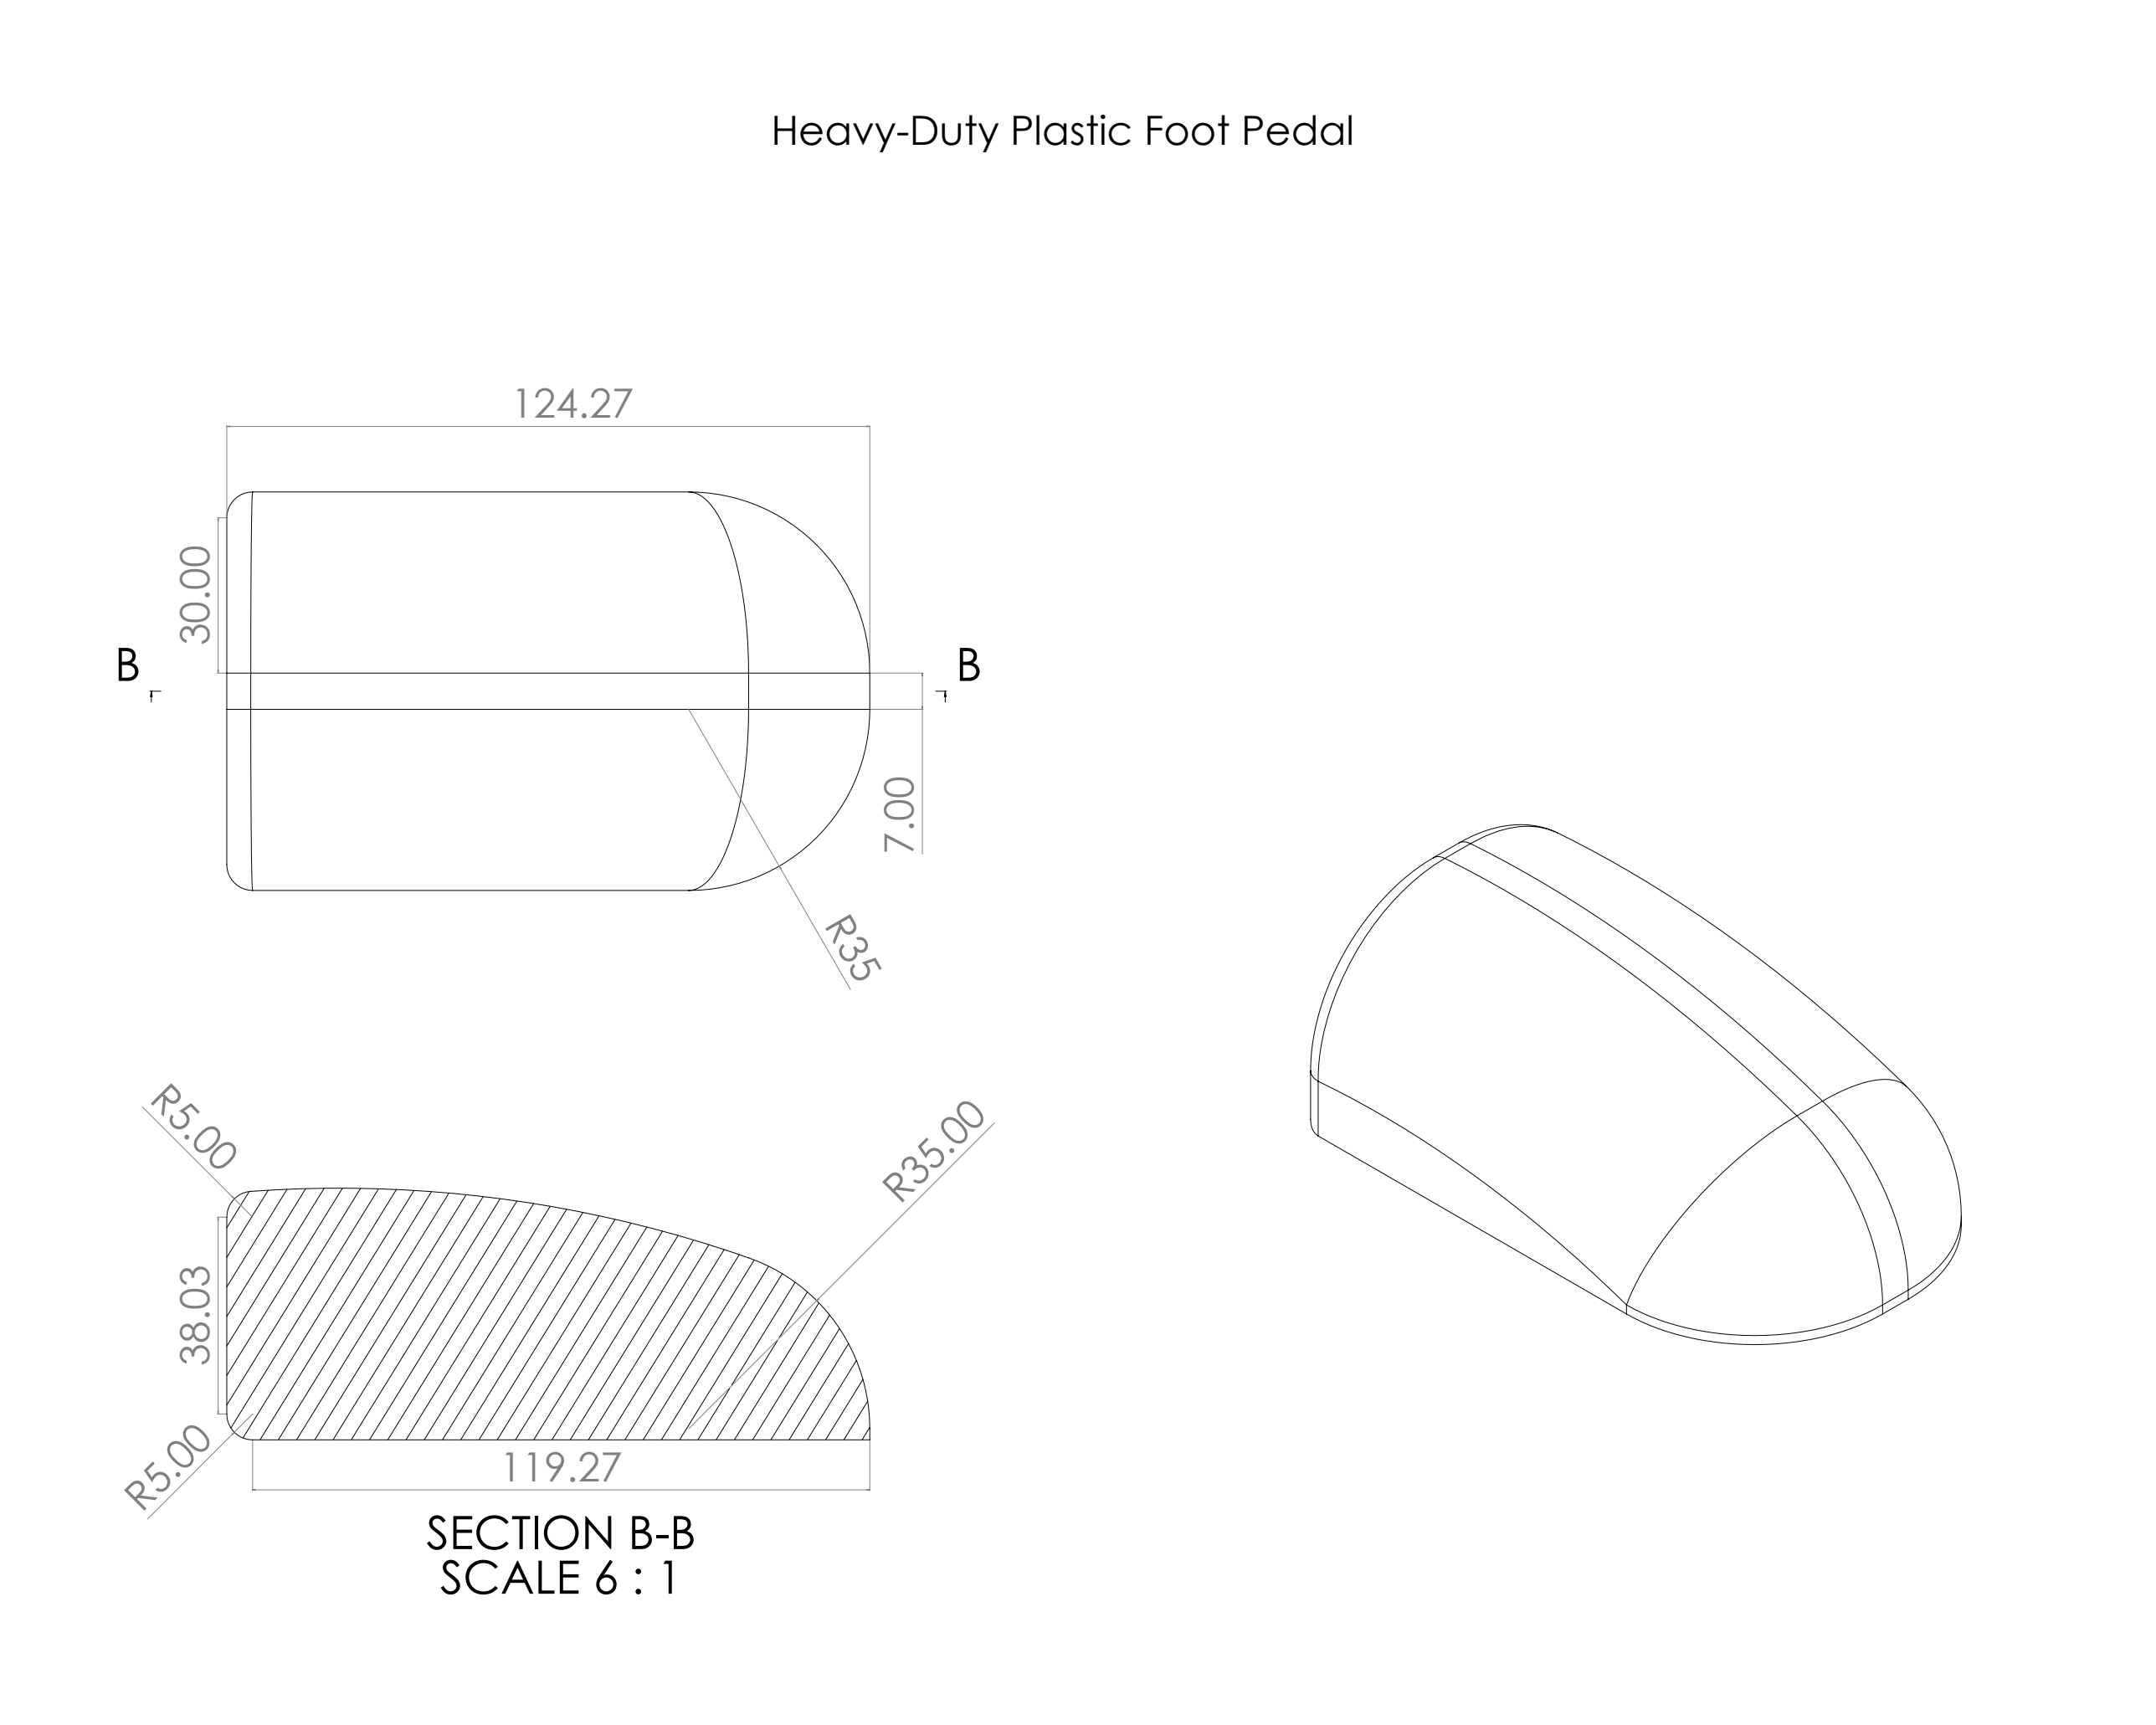
ISO-10303-21;
HEADER;
FILE_DESCRIPTION (('STEP AP214'),
    '1' );
FILE_NAME ('Heavy-Duty Plastic Foot Pedal.step',
    '2026-10-25T20:52:49',
    ( '' ),
    ( '' ),
    'SwSTEP 2.0',
    'SolidWorks 2025',
    '' );
FILE_SCHEMA (( 'AUTOMOTIVE_DESIGN' ));
ENDSEC;

DATA;
#100=CARTESIAN_POINT ( 'NONE',  ( -43.48489315514932230, -254.2578831974578009, -445.7297432066186502 ) ) ;
#247=CARTESIAN_POINT ( 'NONE',  ( -48.18343439339132317, -269.7948820652942459, -438.7219023890238532 ) ) ;
#724=CARTESIAN_POINT ( 'NONE',  ( -48.18343439339130896, -254.0284636146130595, -457.8806065563920242 ) ) ;
#953=CARTESIAN_POINT ( 'NONE',  ( -43.47555712338063927, -255.2612651217553434, -494.0498651529597964 ) ) ;
#1034=CARTESIAN_POINT ( 'NONE',  ( -43.21052124919093984, -280.7960701182722687, -430.6442049081570644 ) ) ;
#1357=CARTESIAN_POINT ( 'NONE',  ( -26.41588298435790350, -486.4924983417995463, -430.6442049081568939 ) ) ;
#1400=CARTESIAN_POINT ( 'NONE',  ( -48.18343439339133027, -283.1093320178188151, -502.6442049081569508 ) ) ;
#1471=DIRECTION ( 'NONE',  ( 0.000000000000000000, 0.000000000000000000, 1.000000000000000000 ) ) ;
#1481=CARTESIAN_POINT ( 'NONE',  ( -43.53110651506508333, -249.2076723177077042, -456.5898888690692843 ) ) ;
#1725=CARTESIAN_POINT ( 'NONE',  ( -43.30989527892933921, -271.8033297790818779, -432.4918912919293916 ) ) ;
#1867=DIRECTION ( 'NONE',  ( 1.000000000000000000, 0.000000000000000000, -0.000000000000000000 ) ) ;
#2208=CARTESIAN_POINT ( 'NONE',  ( -48.18343439340325318, -266.1601729329962609, -435.2001266877076660 ) ) ;
#2229=CARTESIAN_POINT ( 'NONE',  ( -48.18343439339130896, -269.7890444396779230, -499.6173591251650237 ) ) ;
#2316=ADVANCED_BREP_SHAPE_REPRESENTATION ( '', ( #28963, #18940 ), #47644 ) ;
#2670=CARTESIAN_POINT ( 'NONE',  ( -48.18343439339131606, -275.1386486105624272, -431.6459793673298009 ) ) ;
#2690=CARTESIAN_POINT ( 'NONE',  ( -48.18343439339133027, -253.8127106430751496, -479.5013660720742905 ) ) ;
#2709=CARTESIAN_POINT ( 'NONE',  ( 41.08708295871279859, -293.9068999365417199, -472.6442049081569508 ) ) ;
#2893=CARTESIAN_POINT ( 'NONE',  ( 76.08708295871279859, -296.0521521680024080, -430.6442049081568939 ) ) ;
#2981=VERTEX_POINT ( 'NONE', #15532 ) ;
#3072=ADVANCED_FACE ( 'NONE', ( #81317 ), #16463, .T. ) ;
#3125=CARTESIAN_POINT ( 'NONE',  ( -48.18343439339133027, -272.4879030626730696, -437.5575391234876861 ) ) ;
#3143=CARTESIAN_POINT ( 'NONE',  ( -43.32092956878232570, -270.7650335506043007, -505.4258654641533326 ) ) ;
#3207=CARTESIAN_POINT ( 'NONE',  ( -43.32098233076673921, -270.7600516457314939, -505.4240078839325179 ) ) ;
#3599=CARTESIAN_POINT ( 'NONE',  ( -48.18343439339138001, -283.1093320178187582, -430.6442049081568371 ) ) ;
#3617=CARTESIAN_POINT ( 'NONE',  ( -48.18343439339133027, -264.4312075782656279, -496.1714326515607922 ) ) ;
#3619=CARTESIAN_POINT ( 'NONE',  ( -48.18343439339134449, -254.0547856900766703, -480.4587914081814688 ) ) ;
#3743=CARTESIAN_POINT ( 'NONE',  ( -43.18343439339132317, -296.0521521680024080, -430.6442049081568939 ) ) ;
#3769=CARTESIAN_POINT ( 'NONE',  ( -43.53109889459130954, -249.2085213603784268, -456.5866734977748251 ) ) ;
#3844=CARTESIAN_POINT ( 'NONE',  ( -48.18343439339133027, -253.0206516614774728, -465.6442049081569508 ) ) ;
#3935=FACE_OUTER_BOUND ( 'NONE', #80868, .T. ) ;
#3953=CARTESIAN_POINT ( 'NONE',  ( -48.18343439339133027, -293.9810843561368756, -505.5731370962914752 ) ) ;
#3993=EDGE_CURVE ( 'NONE', #34997, #58159, #35812, .T. ) ;
#4087=CARTESIAN_POINT ( 'NONE',  ( -48.18343439339133027, -276.2959221541308352, -501.8817130774843918 ) ) ;
#4229=CARTESIAN_POINT ( 'NONE',  ( -48.18343439339133027, -253.0206516614774159, -465.6442049081569508 ) ) ;
#4302=LINE ( 'NONE', #17587, #66830 ) ;
#4542=CARTESIAN_POINT ( 'NONE',  ( -48.18343439339133027, -249.2745803555438897, -480.5695237573682448 ) ) ;
#4690=CARTESIAN_POINT ( 'NONE',  ( -48.18343439339135159, -250.7819852860406229, -452.8786885270839093 ) ) ;
#4904=ORIENTED_EDGE ( 'NONE', *, *, #49759, .T. ) ;
#5021=CARTESIAN_POINT ( 'NONE',  ( -48.18343439339133027, -251.4422407193385709, -487.0093695598080785 ) ) ;
#5179=CARTESIAN_POINT ( 'NONE',  ( -48.18343439339133027, -259.2349860072159800, -447.3766206888376473 ) ) ;
#5211=AXIS2_PLACEMENT_3D ( 'NONE', #50876, #15355, #79758 ) ;
#5499=CARTESIAN_POINT ( 'NONE',  ( -43.54160339317981965, -248.0334966641277106, -474.9586982258124408 ) ) ;
#5961=DIRECTION ( 'NONE',  ( 0.000000000000000000, 1.000000000000000000, -0.000000000000000000 ) ) ;
#6024=LINE ( 'NONE', #86004, #72995 ) ;
#6089=ORIENTED_EDGE ( 'NONE', *, *, #8182, .F. ) ;
#6470=CARTESIAN_POINT ( 'NONE',  ( 52.66432107828247666, -260.8771019122912094, -430.6442049081568939 ) ) ;
#6500=DIRECTION ( 'NONE',  ( 0.000000000000000000, 0.000000000000000000, 1.000000000000000000 ) ) ;
#6900=CARTESIAN_POINT ( 'NONE',  ( -48.18343439339133027, -253.0206516614774728, -465.6442049081569508 ) ) ;
#7204=CARTESIAN_POINT ( 'NONE',  ( -43.53359761804701833, -248.9297984573114206, -457.6993533439309090 ) ) ;
#7254=ORIENTED_EDGE ( 'NONE', *, *, #66289, .T. ) ;
#7346=CARTESIAN_POINT ( 'NONE',  ( -48.18343439339133027, -279.1637174034430018, -435.8377362501374819 ) ) ;
#7407=ADVANCED_FACE ( 'NONE', ( #36001 ), #88022, .F. ) ;
#7588=DIRECTION ( 'NONE',  ( 0.000000000000000000, 1.000000000000000000, -0.000000000000000000 ) ) ;
#7653=CARTESIAN_POINT ( 'NONE',  ( -43.36971919400434672, -266.0673380770966219, -435.0464150650843180 ) ) ;
#7803=CARTESIAN_POINT ( 'NONE',  ( -48.18343439339131606, -268.0651010539579033, -439.6569430059153092 ) ) ;
#7831=EDGE_CURVE ( 'NONE', #89245, #73999, #37835, .T. ) ;
#8036=CARTESIAN_POINT ( 'NONE',  ( -43.39876772438888963, -263.1881392940089199, -501.4585950967926919 ) ) ;
#8182=EDGE_CURVE ( 'NONE', #87518, #58102, #33614, .T. ) ;
#8279=CARTESIAN_POINT ( 'NONE',  ( -48.18343439339133027, -263.2279375583058822, -443.0391293176500085 ) ) ;
#8379=DIRECTION ( 'NONE',  ( 0.000000000000000000, 1.000000000000000000, 0.000000000000000000 ) ) ;
#8460=ORIENTED_EDGE ( 'NONE', *, *, #28009, .F. ) ;
#8475=CARTESIAN_POINT ( 'NONE',  ( -48.18343439339133027, -283.1093320178187582, -435.6442049081568939 ) ) ;
#8499=CARTESIAN_POINT ( 'NONE',  ( -48.18343439339133027, -268.0622923073750030, -498.6988577444290627 ) ) ;
#8502=CARTESIAN_POINT ( 'NONE',  ( -48.18343439339133027, -296.0521521680024080, -507.6442049081570076 ) ) ;
#8798=ORIENTED_EDGE ( 'NONE', *, *, #42527, .T. ) ;
#8817=CARTESIAN_POINT ( 'NONE',  ( -48.18343439339132317, -274.0269255681727145, -431.9367980400547253 ) ) ;
#8831=CARTESIAN_POINT ( 'NONE',  ( -43.18343439339132317, -283.1093320178187582, -502.6442049081569508 ) ) ;
#9276=CARTESIAN_POINT ( 'NONE',  ( -48.18343439339133027, -269.7948820652890731, -438.7219023889692835 ) ) ;
#9290=DIRECTION ( 'NONE',  ( 0.000000000000000000, 0.000000000000000000, 1.000000000000000000 ) ) ;
#9339=DIRECTION ( 'NONE',  ( 0.000000000000000000, 0.000000000000000000, 1.000000000000000000 ) ) ;
#9763=CARTESIAN_POINT ( 'NONE',  ( -43.43092116352006826, -259.9338699230254406, -439.2716167192226067 ) ) ;
#10045=VERTEX_POINT ( 'NONE', #56044 ) ;
#10215=CARTESIAN_POINT ( 'NONE',  ( -48.18343439339133027, -273.4097382618878100, -437.2279360942110884 ) ) ;
#10234=CARTESIAN_POINT ( 'NONE',  ( -48.18343439339133738, -283.1093320178188151, -507.6442049081570076 ) ) ;
#10236=CARTESIAN_POINT ( 'NONE',  ( -48.18343439339132317, -257.0657538259918056, -487.6787901984505993 ) ) ;
#10296=CARTESIAN_POINT ( 'NONE',  ( -43.18343439339132317, -296.0521521680024080, -507.6442049081570076 ) ) ;
#10561=DIRECTION ( 'NONE',  ( 0.000000000000000000, 0.000000000000000000, 1.000000000000000000 ) ) ;
#10566=CARTESIAN_POINT ( 'NONE',  ( -43.18343439339132317, -296.0521521680024080, -507.6442049081570076 ) ) ;
#10684=CARTESIAN_POINT ( 'NONE',  ( -48.18343439336744183, -267.6629864561588761, -434.3825974374845487 ) ) ;
#10848=CARTESIAN_POINT ( 'NONE',  ( -48.18343439339133027, -249.2485278041818901, -457.7706553364274100 ) ) ;
#10891=CARTESIAN_POINT ( 'NONE',  ( -26.41588298435790350, -486.4924983417995463, -472.6442049081569508 ) ) ;
#11180=CARTESIAN_POINT ( 'NONE',  ( -48.18343439339133027, -257.8434817577961553, -488.9450021219734595 ) ) ;
#11251=CARTESIAN_POINT ( 'NONE',  ( -43.30935424508157183, -271.8540379715383324, -505.8138214194312923 ) ) ;
#11332=CARTESIAN_POINT ( 'NONE',  ( -43.48485865067390677, -254.2615844090929045, -445.7244014337675253 ) ) ;
#11407=DIRECTION ( 'NONE',  ( 1.000000000000000000, 2.720159063138535749E-15, 0.000000000000000000 ) ) ;
#11540=ORIENTED_EDGE ( 'NONE', *, *, #43526, .F. ) ;
#11595=ORIENTED_EDGE ( 'NONE', *, *, #61799, .F. ) ;
#11665=ORIENTED_EDGE ( 'NONE', *, *, #83215, .T. ) ;
#11792=CARTESIAN_POINT ( 'NONE',  ( -48.18343439339133027, -248.3668650810685676, -465.6442049081568371 ) ) ;
#11902=PLANE ( 'NONE',  #52058 ) ;
#12001=ORIENTED_EDGE ( 'NONE', *, *, #33757, .T. ) ;
#12115=CARTESIAN_POINT ( 'NONE',  ( -43.53450001092989652, -248.8289484981847863, -480.0790493083237607 ) ) ;
#12180=CARTESIAN_POINT ( 'NONE',  ( -43.49890293645135841, -252.7466870590830865, -490.1793782242883708 ) ) ;
#12264=CARTESIAN_POINT ( 'NONE',  ( -43.52658375460264750, -249.7100083083012692, -454.9363245936367548 ) ) ;
#12597=DIRECTION ( 'NONE',  ( 0.000000000000000000, 0.000000000000000000, 1.000000000000000000 ) ) ;
#12629=ORIENTED_EDGE ( 'NONE', *, *, #43955, .F. ) ;
#12885=ORIENTED_EDGE ( 'NONE', *, *, #48330, .F. ) ;
#12974=ORIENTED_EDGE ( 'NONE', *, *, #37852, .F. ) ;
#13029=AXIS2_PLACEMENT_3D ( 'NONE', #44407, #79937, #16464 ) ;
#13060=CARTESIAN_POINT ( 'NONE',  ( 41.08708295871279859, -293.9068999365417199, -472.6442049081569508 ) ) ;
#13079=CARTESIAN_POINT ( 'NONE',  ( -48.18343439338445933, -248.5908816770286762, -477.2051880179521959 ) ) ;
#13333=VECTOR ( 'NONE', #26325, 1000.000000000000000 ) ;
#13470=ADVANCED_FACE ( 'NONE', ( #85701 ), #71045, .T. ) ;
#13582=ORIENTED_EDGE ( 'NONE', *, *, #62145, .F. ) ;
#13624=CARTESIAN_POINT ( 'NONE',  ( 76.08708295871279859, -296.0521521680024080, -472.6442049081569508 ) ) ;
#13813=( LENGTH_UNIT ( ) NAMED_UNIT ( * ) SI_UNIT ( .MILLI., .METRE. ) );
#13848=CARTESIAN_POINT ( 'NONE',  ( -43.37481164453355120, -265.5671965738019367, -435.3290497496450371 ) ) ;
#13871=CARTESIAN_POINT ( 'NONE',  ( -43.18343439339132317, -291.0521521680024080, -430.6442049081568939 ) ) ;
#14003=CARTESIAN_POINT ( 'NONE',  ( -48.18343439339130896, -259.5409938266968197, -446.9856792133138583 ) ) ;
#14206=DIRECTION ( 'NONE',  ( -0.000000000000000000, 1.000000000000000000, -0.000000000000000000 ) ) ;
#14230=AXIS2_PLACEMENT_3D ( 'NONE', #31675, #81847, #15601 ) ;
#14261=CYLINDRICAL_SURFACE ( 'NONE', #29226, 35.00000000000002842 ) ;
#14693=CARTESIAN_POINT ( 'NONE',  ( 41.08708295871279859, -293.9068999365417199, -430.6442049081568939 ) ) ;
#14929=CARTESIAN_POINT ( 'NONE',  ( -48.18343439339133027, -266.7963633757954085, -440.4292507799816576 ) ) ;
#15126=FACE_OUTER_BOUND ( 'NONE', #63166, .T. ) ;
#15204=ORIENTED_EDGE ( 'NONE', *, *, #7831, .T. ) ;
#15234=CARTESIAN_POINT ( 'NONE',  ( -43.48180805801840165, -254.5884423091092117, -445.2610164474263001 ) ) ;
#15355=DIRECTION ( 'NONE',  ( 0.000000000000000000, 0.000000000000000000, 1.000000000000000000 ) ) ;
#15382=CARTESIAN_POINT ( 'NONE',  ( -48.18343439339134449, -276.7382201398751249, -436.3198488720590262 ) ) ;
#15532=CARTESIAN_POINT ( 'NONE',  ( 76.08708295871279859, -296.0521521680024080, -472.6442049081569508 ) ) ;
#15539=MECHANICAL_DESIGN_GEOMETRIC_PRESENTATION_REPRESENTATION('',(#48848),#88107);
#15601=DIRECTION ( 'NONE',  ( -0.3307782319877045629, -0.9437085149785860994, 0.000000000000000000 ) ) ;
#15613=CARTESIAN_POINT ( 'NONE',  ( -43.43026024688149533, -259.9949877806594714, -498.9966730678170279 ) ) ;
#15811=DIRECTION ( 'NONE',  ( 0.000000000000000000, -0.000000000000000000, 1.000000000000000000 ) ) ;
#15920=EDGE_LOOP ( 'NONE', ( #24151, #50514, #36761, #12885 ) ) ;
#16404=CARTESIAN_POINT ( 'NONE',  ( -48.18343439339133027, -275.2947406849283425, -436.6688341897090595 ) ) ;
#16463=CYLINDRICAL_SURFACE ( 'NONE', #70181, 5.000000000000004441 ) ;
#16464=DIRECTION ( 'NONE',  ( 1.000000000000000000, 0.000000000000000000, 0.000000000000000000 ) ) ;
#16486=VECTOR ( 'NONE', #91022, 1000.000000000000000 ) ;
#16611=CARTESIAN_POINT ( 'NONE',  ( 76.08708295871279859, -296.0521521680024080, -465.6442049081569508 ) ) ;
#16758=CARTESIAN_POINT ( 'NONE',  ( -43.18343439339132317, -296.0521521680024080, -430.6442049081568939 ) ) ;
#16846=ORIENTED_EDGE ( 'NONE', *, *, #91011, .T. ) ;
#16867=CARTESIAN_POINT ( 'NONE',  ( -43.29218995563469718, -273.4472827993805595, -431.9929295280254564 ) ) ;
#17052=ORIENTED_EDGE ( 'NONE', *, *, #50609, .F. ) ;
#17349=CARTESIAN_POINT ( 'NONE',  ( -43.26778476368559012, -275.6832172112468129, -431.4324561993768157 ) ) ;
#17434=CARTESIAN_POINT ( 'NONE',  ( -43.23637629196743148, -278.5210525055342146, -507.4181868956659969 ) ) ;
#17513=CARTESIAN_POINT ( 'NONE',  ( -43.18343439339132317, -283.1093320178187582, -430.6442049081568939 ) ) ;
#17538=ORIENTED_EDGE ( 'NONE', *, *, #64655, .F. ) ;
#17587=CARTESIAN_POINT ( 'NONE',  ( 41.08708295871279859, -270.5084069056321141, -430.6442049081568939 ) ) ;
#17636=EDGE_LOOP ( 'NONE', ( #81351, #74447, #32798, #66890 ) ) ;
#17805=CARTESIAN_POINT ( 'NONE',  ( -48.18343439339133027, -279.1637174034569284, -435.8377362500897902 ) ) ;
#17825=CARTESIAN_POINT ( 'NONE',  ( -48.18343439339133027, -269.7890444396509793, -499.6173591253298127 ) ) ;
#17828=CARTESIAN_POINT ( 'NONE',  ( -48.18343439339133027, -262.5501068226030839, -494.5729214566502492 ) ) ;
#17892=CARTESIAN_POINT ( 'NONE',  ( -43.47559602926583722, -255.2571177548196317, -494.0444526766419813 ) ) ;
#18050=( LENGTH_UNIT ( ) NAMED_UNIT ( * ) SI_UNIT ( .MILLI., .METRE. ) );
#18213=ORIENTED_EDGE ( 'NONE', *, *, #28676, .T. ) ;
#18232=EDGE_LOOP ( 'NONE', ( #7254, #18926, #87600, #85867, #69916, #62240 ) ) ;
#18283=CARTESIAN_POINT ( 'NONE',  ( -48.18343439339133027, -266.0193969580721500, -497.3422536412488739 ) ) ;
#18346=SPHERICAL_SURFACE ( 'NONE', #26517, 35.00000000000000000 ) ;
#18358=CARTESIAN_POINT ( 'NONE',  ( 76.08708295871279859, -293.9068999365417199, -472.6442049081569508 ) ) ;
#18427=CARTESIAN_POINT ( 'NONE',  ( -48.18343439339133027, -256.0722001993605090, -452.3316844813846842 ) ) ;
#18706=CIRCLE ( 'NONE', #30804, 35.00000000000002842 ) ;
#18762=CARTESIAN_POINT ( 'NONE',  ( -48.18343439339133027, -253.8127106430984554, -479.5013660720755979 ) ) ;
#18832=CARTESIAN_POINT ( 'NONE',  ( -43.18343439339132317, -283.1093320178187582, -507.6442049081570076 ) ) ;
#18843=EDGE_LOOP ( 'NONE', ( #20360, #26128, #11665, #73887 ) ) ;
#18912=CYLINDRICAL_SURFACE ( 'NONE', #19457, 5.000000000000004441 ) ;
#18926=ORIENTED_EDGE ( 'NONE', *, *, #77324, .T. ) ;
#18940=AXIS2_PLACEMENT_3D ( 'NONE', #90959, #40773, #33703 ) ;
#19002=ORIENTED_EDGE ( 'NONE', *, *, #73107, .F. ) ;
#19011=VECTOR ( 'NONE', #52807, 1000.000000000000000 ) ;
#19035=EDGE_LOOP ( 'NONE', ( #50833, #50359, #8798, #18213 ) ) ;
#19224=CYLINDRICAL_SURFACE ( 'NONE', #81359, 35.00000000000002842 ) ;
#19288=CARTESIAN_POINT ( 'NONE',  ( -43.53335921173260914, -248.9562857179395508, -480.6412943097532207 ) ) ;
#19366=CARTESIAN_POINT ( 'NONE',  ( -43.50953176532448907, -251.5913190049807611, -450.1129310769470067 ) ) ;
#19376=ORIENTED_EDGE ( 'NONE', *, *, #83986, .F. ) ;
#19457=AXIS2_PLACEMENT_3D ( 'NONE', #68636, #47286, #83282 ) ;
#19519=EDGE_LOOP ( 'NONE', ( #82802, #11595, #56209, #58303 ) ) ;
#19682=CARTESIAN_POINT ( 'NONE',  ( -43.53082020000776708, -249.2392102346787510, -481.7612224915185948 ) ) ;
#19727=DIRECTION ( 'NONE',  ( -0.000000000000000000, -0.000000000000000000, -1.000000000000000000 ) ) ;
#20156=AXIS2_PLACEMENT_3D ( 'NONE', #72886, #24078, #45847 ) ;
#20191=VERTEX_POINT ( 'NONE', #22545 ) ;
#20360=ORIENTED_EDGE ( 'NONE', *, *, #64884, .T. ) ;
#20636=CARTESIAN_POINT ( 'NONE',  ( -48.18343439338621437, -252.7258303143705120, -489.5392129326988311 ) ) ;
#20941=CARTESIAN_POINT ( 'NONE',  ( -43.43097417488520762, -259.9284170800161178, -439.2763949627545799 ) ) ;
#21156=AXIS2_PLACEMENT_3D ( 'NONE', #13871, #42723, #71168 ) ;
#21638=CIRCLE ( 'NONE', #50361, 5.000000000000004441 ) ;
#21853=ORIENTED_EDGE ( 'NONE', *, *, #61799, .T. ) ;
#21989=EDGE_LOOP ( 'NONE', ( #4904, #67175, #12001, #84021 ) ) ;
#22034=CARTESIAN_POINT ( 'NONE',  ( -48.18343439339133027, -276.2535042660555860, -436.4286699060131696 ) ) ;
#22185=ORIENTED_EDGE ( 'NONE', *, *, #83488, .T. ) ;
#22202=LINE ( 'NONE', #79960, #68394 ) ;
#22256=CARTESIAN_POINT ( 'NONE',  ( -48.18343439339133027, -263.2803689378613399, -495.2320347593685597 ) ) ;
#22260=DIRECTION ( 'NONE',  ( -0.000000000000000000, 0.000000000000000000, -1.000000000000000000 ) ) ;
#22545=CARTESIAN_POINT ( 'NONE',  ( 41.08708295871279859, -296.0521521680024080, -430.6442049081568939 ) ) ;
#22704=CARTESIAN_POINT ( 'NONE',  ( -43.49337173925265887, -253.3453352546504220, -491.1732795760416366 ) ) ;
#22707=CARTESIAN_POINT ( 'NONE',  ( -48.18343439339133027, -248.4123448508205172, -430.6442049081568939 ) ) ;
#22861=EDGE_CURVE ( 'NONE', #64125, #20191, #29124, .T. ) ;
#22909=DIRECTION ( 'NONE',  ( 0.000000000000000000, 0.000000000000000000, 1.000000000000000000 ) ) ;
#22943=CARTESIAN_POINT ( 'NONE',  ( -48.18343439339131606, -253.2159931059841256, -461.7098312862314629 ) ) ;
#23175=CARTESIAN_POINT ( 'NONE',  ( -48.18343439339476930, -260.1500860263135451, -498.8200089662520327 ) ) ;
#23250=DIRECTION ( 'NONE',  ( 0.000000000000000000, 0.000000000000000000, -1.000000000000000000 ) ) ;
#23371=ORIENTED_EDGE ( 'NONE', *, *, #3993, .F. ) ;
#23533=CARTESIAN_POINT ( 'NONE',  ( -48.18343439339133738, -256.1235685800110673, -485.9512705677856275 ) ) ;
#23842=CARTESIAN_POINT ( 'NONE',  ( 41.08708295871279859, -296.0521521680024080, -465.6442049081569508 ) ) ;
#23858=CARTESIAN_POINT ( 'NONE',  ( 41.08708295871279859, -296.0521521680024080, -507.6442049081570076 ) ) ;
#23967=CARTESIAN_POINT ( 'NONE',  ( -43.38476897654369679, -264.5837039706560745, -435.9172296759396659 ) ) ;
#24078=DIRECTION ( 'NONE',  ( 0.000000000000000000, 1.000000000000000000, 0.000000000000000000 ) ) ;
#24151=ORIENTED_EDGE ( 'NONE', *, *, #39969, .F. ) ;
#24195=DIRECTION ( 'NONE',  ( -0.000000000000000000, -0.000000000000000000, -1.000000000000000000 ) ) ;
#24428=CARTESIAN_POINT ( 'NONE',  ( -43.27399328867051054, -275.1182110581578968, -431.5594140723246142 ) ) ;
#24451=CARTESIAN_POINT ( 'NONE',  ( -48.18343439339133027, -254.1872365014070567, -480.9328361744650806 ) ) ;
#24763=CIRCLE ( 'NONE', #83748, 35.00000000000002842 ) ;
#24911=CARTESIAN_POINT ( 'NONE',  ( -48.18343439338274692, -265.6649765806887444, -435.4852526219743822 ) ) ;
#24931=CARTESIAN_POINT ( 'NONE',  ( -48.18343439341186496, -262.8409108322527459, -500.9583777586229871 ) ) ;
#24982=EDGE_LOOP ( 'NONE', ( #47654, #89532, #19002, #26723 ) ) ;
#25148=DIRECTION ( 'NONE',  ( 0.000000000000000000, 1.000000000000000000, -0.000000000000000000 ) ) ;
#25194=ORIENTED_EDGE ( 'NONE', *, *, #33757, .F. ) ;
#25349=EDGE_CURVE ( 'NONE', #10045, #89245, #65738, .T. ) ;
#25365=CARTESIAN_POINT ( 'NONE',  ( -48.18343439340851830, -256.9335312097066435, -442.7126937774146427 ) ) ;
#25382=CARTESIAN_POINT ( 'NONE',  ( -48.18343439338961076, -261.4749445206144856, -499.9176714739165277 ) ) ;
#25384=CARTESIAN_POINT ( 'NONE',  ( -48.18343439339133027, -283.1093320178187582, -502.6442049081569508 ) ) ;
#25530=CARTESIAN_POINT ( 'NONE',  ( -48.18343439339133027, -252.9280701297265637, -448.2498469311837539 ) ) ;
#25617=CARTESIAN_POINT ( 'NONE',  ( -43.54160339317392214, -248.0334966641272842, -472.6442049081569508 ) ) ;
#25732=CARTESIAN_POINT ( 'NONE',  ( -43.18343439339132317, -248.4123448508205172, -502.6442049081569508 ) ) ;
#25842=CARTESIAN_POINT ( 'NONE',  ( -43.51344012988974441, -251.1608963058792199, -487.1372761508537224 ) ) ;
#25843=CARTESIAN_POINT ( 'NONE',  ( -48.18343439339133027, -296.0521521680024080, -430.6442049081568939 ) ) ;
#25908=CARTESIAN_POINT ( 'NONE',  ( -43.50152060878402693, -252.4623848617872852, -489.6796197559582424 ) ) ;
#25990=CARTESIAN_POINT ( 'NONE',  ( -48.18343439339133027, -255.1274621574002310, -454.6030467723235802 ) ) ;
#26128=ORIENTED_EDGE ( 'NONE', *, *, #69089, .T. ) ;
#26284=AXIS2_PLACEMENT_3D ( 'NONE', #14693, #29360, #35047 ) ;
#26325=DIRECTION ( 'NONE',  ( 1.000000000000000000, 0.000000000000000000, 0.000000000000000000 ) ) ;
#26362=ORIENTED_EDGE ( 'NONE', *, *, #67205, .F. ) ;
#26397=CARTESIAN_POINT ( 'NONE',  ( -43.40350038011558809, -262.7128720674827491, -501.1256881030387262 ) ) ;
#26478=CARTESIAN_POINT ( 'NONE',  ( -48.18343439339133027, -253.2159931059258042, -461.7098312862245280 ) ) ;
#26517=AXIS2_PLACEMENT_3D ( 'NONE', #32087, #39623, #54786 ) ;
#26556=CARTESIAN_POINT ( 'NONE',  ( -26.41588298435790350, -486.4924983417995463, -507.6442049081570076 ) ) ;
#26661=CARTESIAN_POINT ( 'NONE',  ( -46.11236658152585477, -296.0521521680024080, -507.6442049081570076 ) ) ;
#26723=ORIENTED_EDGE ( 'NONE', *, *, #42150, .F. ) ;
#26798=CARTESIAN_POINT ( 'NONE',  ( -48.18343439339133027, -250.5789762915055405, -484.9196478893141489 ) ) ;
#26799=CARTESIAN_POINT ( 'NONE',  ( 41.08708295871279859, -296.0521521680024080, -465.6442049081569508 ) ) ;
#26941=CARTESIAN_POINT ( 'NONE',  ( -48.18343439339133027, -253.0206516619178956, -463.6604981723916694 ) ) ;
#27132=CYLINDRICAL_SURFACE ( 'NONE', #21156, 5.000000000000004441 ) ;
#27264=CARTESIAN_POINT ( 'NONE',  ( -48.18343439339133738, -249.5520599237212593, -481.6766596038578427 ) ) ;
#27627=CYLINDRICAL_SURFACE ( 'NONE', #52977, 5.000000000000004441 ) ;
#27718=AXIS2_PLACEMENT_3D ( 'NONE', #32219, #1471, #84263 ) ;
#27878=EDGE_CURVE ( 'NONE', #33307, #86528, #29133, .T. ) ;
#28009=EDGE_CURVE ( 'NONE', #33307, #47563, #39636, .T. ) ;
#28029=( NAMED_UNIT ( * ) PLANE_ANGLE_UNIT ( ) SI_UNIT ( $, .RADIAN. ) );
#28516=CARTESIAN_POINT ( 'NONE',  ( -43.35418436979174572, -267.5839012688533671, -434.2375725762524326 ) ) ;
#28567=PRODUCT ( 'Heavy-Duty Plastic Foot Pedal', 'Heavy-Duty Plastic Foot Pedal', '', ( #46386 ) ) ;
#28676=EDGE_CURVE ( 'NONE', #40166, #73999, #45041, .T. ) ;
#28911=ORIENTED_EDGE ( 'NONE', *, *, #68922, .T. ) ;
#28963=MANIFOLD_SOLID_BREP ( 'Fillet12', #46108 ) ;
#28979=CARTESIAN_POINT ( 'NONE',  ( -43.47202469644348355, -255.6311900920820790, -443.8813325122532660 ) ) ;
#29074=ORIENTED_EDGE ( 'NONE', *, *, #25349, .T. ) ;
#29124=CIRCLE ( 'NONE', #44240, 35.00000000000002842 ) ;
#29130=CARTESIAN_POINT ( 'NONE',  ( -48.18343439339133027, -258.3625464905466629, -448.5700876443984839 ) ) ;
#29133=CIRCLE ( 'NONE', #44185, 204.0731808058633590 ) ;
#29226=AXIS2_PLACEMENT_3D ( 'NONE', #43119, #7588, #50692 ) ;
#29313=CARTESIAN_POINT ( 'NONE',  ( -43.18343439339132317, -253.0206516614774159, -465.6442049081569508 ) ) ;
#29360=DIRECTION ( 'NONE',  ( -0.000000000000000000, -0.000000000000000000, -1.000000000000000000 ) ) ;
#29454=CARTESIAN_POINT ( 'NONE',  ( -43.33278562674490075, -269.6489459241407758, -433.2630959494377976 ) ) ;
#29564=ADVANCED_FACE ( 'NONE', ( #30709 ), #88909, .T. ) ;
#29640=TOROIDAL_SURFACE ( 'NONE', #13029, 204.0731808058633590, 35.00000000000000000 ) ;
#29831=CARTESIAN_POINT ( 'NONE',  ( -43.40344324565903378, -262.7186194818502827, -501.1297839416856164 ) ) ;
#30030=SHAPE_REPRESENTATION ( 'Heavy-Duty Plastic Foot Pedal', ( #18940 ), #47644 ) ;
#30061=CARTESIAN_POINT ( 'NONE',  ( -48.18343439339133027, -271.5660680172725847, -437.8871425252946210 ) ) ;
#30185=ORIENTED_EDGE ( 'NONE', *, *, #50609, .T. ) ;
#30245=VERTEX_POINT ( 'NONE', #18358 ) ;
#30287=CARTESIAN_POINT ( 'NONE',  ( -48.18343439338453749, -278.5340725472075860, -507.3671153682459476 ) ) ;
#30544=EDGE_CURVE ( 'NONE', #51410, #47679, #36554, .T. ) ;
#30612=CARTESIAN_POINT ( 'NONE',  ( -43.23650051345222067, -278.5104573893707993, -430.8699914737978816 ) ) ;
#30709=FACE_OUTER_BOUND ( 'NONE', #71954, .T. ) ;
#30804=AXIS2_PLACEMENT_3D ( 'NONE', #13060, #92088, #49021 ) ;
#30930=VERTEX_POINT ( 'NONE', #36758 ) ;
#31112=CARTESIAN_POINT ( 'NONE',  ( -48.18343439339133027, -276.2959221541210582, -501.8817130775132682 ) ) ;
#31463=ADVANCED_FACE ( 'NONE', ( #3935 ), #88338, .F. ) ;
#31549=CARTESIAN_POINT ( 'NONE',  ( -48.18343439339989942, -264.6857882449573935, -436.0815118164402975 ) ) ;
#31571=CARTESIAN_POINT ( 'NONE',  ( -48.18343439339133027, -260.4667269299101804, -492.5001339377540717 ) ) ;
#31675=CARTESIAN_POINT ( 'NONE',  ( 41.08708295871279859, -293.9068999365417199, -465.6442049081569508 ) ) ;
#31694=AXIS2_PLACEMENT_3D ( 'NONE', #45495, #67321, #60679 ) ;
#31747=APPLICATION_CONTEXT ( 'automotive_design' ) ;
#31789=( NAMED_UNIT ( * ) SI_UNIT ( $, .STERADIAN. ) SOLID_ANGLE_UNIT ( ) );
#31799=ORIENTED_EDGE ( 'NONE', *, *, #27878, .T. ) ;
#31975=ORIENTED_EDGE ( 'NONE', *, *, #62639, .F. ) ;
#32005=CARTESIAN_POINT ( 'NONE',  ( -48.18343439339133027, -263.2279375582672856, -443.0391293175771352 ) ) ;
#32025=CARTESIAN_POINT ( 'NONE',  ( -48.18343439343219359, -265.6641742835798823, -502.8827764852874225 ) ) ;
#32087=CARTESIAN_POINT ( 'NONE',  ( 41.08708295871279859, -293.9068999365417199, -465.6442049081569508 ) ) ;
#32114=B_SPLINE_CURVE_WITH_KNOTS ( 'NONE', 3,
 ( #65146, #73156, #7346, #15382, #22034, #43335, #44246, #73618, #30061, #247, #50439, #7803, #36690, #14929, #58946, #8279, #78853, #57101, #14003, #43784, #71777, #29130, #42863, #37159, #66068, #85941, #724, #87794, #22943, #93057, #6900 ),
 .UNSPECIFIED., .F., .F.,
 ( 4, 2, 2, 2, 1, 2, 2, 2, 2, 2, 2, 2, 2, 2, 2, 4 ),
 ( 0.000000000000000000, 0.005913895122008330264, 0.007392368902510404807, 0.008870842683012480218, 0.01182779024401667614, 0.01478473780502087206, 0.01626321158552301166, 0.01774168536602514779, 0.02365558048803392821, 0.02661252804903820046, 0.02809100182954044761, 0.02956947561004270170, 0.03548337073205194009, 0.03844031829305656622, 0.04139726585406118542, 0.04731116097607026422 ),
 .UNSPECIFIED. ) ;
#32149=CARTESIAN_POINT ( 'NONE',  ( -48.18343439339133027, -291.0521521680024080, -435.6442049081568939 ) ) ;
#32219=CARTESIAN_POINT ( 'NONE',  ( 41.08708295871279859, -293.9068999365417199, -472.6442049081569508 ) ) ;
#32229=VECTOR ( 'NONE', #14206, 1000.000000000000000 ) ;
#32486=CARTESIAN_POINT ( 'NONE',  ( -43.18343439339132317, -283.1093320178187582, -430.6442049081568939 ) ) ;
#32504=CARTESIAN_POINT ( 'NONE',  ( -48.18343439339133027, -260.4667269298406040, -492.5001339377689078 ) ) ;
#32506=CARTESIAN_POINT ( 'NONE',  ( -48.18343439339132317, -268.0622923074284358, -498.6988577443486861 ) ) ;
#32575=CARTESIAN_POINT ( 'NONE',  ( -43.27353253609506112, -275.1640841960933699, -506.7538176778678576 ) ) ;
#32585=EDGE_CURVE ( 'NONE', #30930, #86528, #68911, .T. ) ;
#32654=CARTESIAN_POINT ( 'NONE',  ( -48.18343439339648171, -250.1936144431593050, -454.4903112404356307 ) ) ;
#32798=ORIENTED_EDGE ( 'NONE', *, *, #64884, .F. ) ;
#32809=DIRECTION ( 'NONE',  ( -1.000000000000000000, 0.000000000000000000, 0.000000000000000000 ) ) ;
#32827=CARTESIAN_POINT ( 'NONE',  ( 52.66432107828247666, -260.8771019122912094, -465.6442049081569508 ) ) ;
#32958=CARTESIAN_POINT ( 'NONE',  ( -48.18343439339133027, -267.6589013224570976, -503.9656168148090956 ) ) ;
#33020=FACE_OUTER_BOUND ( 'NONE', #66751, .T. ) ;
#33106=CARTESIAN_POINT ( 'NONE',  ( -43.54160339320051065, -248.0334966641291601, -463.3298803830878114 ) ) ;
#33147=ORIENTED_EDGE ( 'NONE', *, *, #30544, .T. ) ;
#33262=ORIENTED_EDGE ( 'NONE', *, *, #30544, .F. ) ;
#33307=VERTEX_POINT ( 'NONE', #91371 ) ;
#33483=CARTESIAN_POINT ( 'NONE',  ( -43.52491939661445031, -249.8948216656541774, -483.9534721554022667 ) ) ;
#33565=CARTESIAN_POINT ( 'NONE',  ( -48.18343439339133027, -256.9970711660205325, -450.6082928460551216 ) ) ;
#33614=( BOUNDED_CURVE ( )  B_SPLINE_CURVE ( 3, ( #32149, #54380, #47259, #3743 ),
 .UNSPECIFIED., .F., .F. ) 
 B_SPLINE_CURVE_WITH_KNOTS ( ( 4, 4 ),
 ( 1.570796326794896558, 3.141592653589793116 ),
 .UNSPECIFIED. ) 
 CURVE ( )  GEOMETRIC_REPRESENTATION_ITEM ( )  RATIONAL_B_SPLINE_CURVE ( ( 1.000000000000000000, 0.8047378541243649375, 0.8047378541243649375, 1.000000000000000000 ) ) 
 REPRESENTATION_ITEM ( '' )  );
#33703=DIRECTION ( 'NONE',  ( 1.000000000000000000, 0.000000000000000000, 0.000000000000000000 ) ) ;
#33757=EDGE_CURVE ( 'NONE', #30930, #42782, #21638, .T. ) ;
#33785=CIRCLE ( 'NONE', #88166, 239.0731808058633590 ) ;
#33902=CARTESIAN_POINT ( 'NONE',  ( -48.18343439339133027, -255.7030234860429516, -485.0668374018911777 ) ) ;
#34054=CARTESIAN_POINT ( 'NONE',  ( -48.18343439338448064, -254.8206355561004273, -445.4195540462232543 ) ) ;
#34133=DIRECTION ( 'NONE',  ( -0.000000000000000000, -0.000000000000000000, -1.000000000000000000 ) ) ;
#34372=CARTESIAN_POINT ( 'NONE',  ( -43.50896817468466793, -251.6512071849481629, -488.1691148443978250 ) ) ;
#34834=CARTESIAN_POINT ( 'NONE',  ( -43.53957993923267367, -248.2613007709077522, -477.2483004490479743 ) ) ;
#34993=ADVANCED_FACE ( 'NONE', ( #46548 ), #75449, .T. ) ;
#34997=VERTEX_POINT ( 'NONE', #32827 ) ;
#35047=DIRECTION ( 'NONE',  ( -1.000000000000000000, 0.000000000000000000, 0.000000000000000000 ) ) ;
#35291=VECTOR ( 'NONE', #24195, 1000.000000000000000 ) ;
#35625=CARTESIAN_POINT ( 'NONE',  ( -43.50955339366421981, -251.5889492418373266, -450.1178138017020274 ) ) ;
#35812=LINE ( 'NONE', #6470, #64130 ) ;
#35902=DIRECTION ( 'NONE',  ( 1.000000000000000000, 0.000000000000000000, 0.000000000000000000 ) ) ;
#36001=FACE_OUTER_BOUND ( 'NONE', #18232, .T. ) ;
#36079=CARTESIAN_POINT ( 'NONE',  ( -43.52509054635434183, -249.8758584012454946, -454.3901068140907000 ) ) ;
#36276=EDGE_CURVE ( 'NONE', #64125, #2981, #61150, .T. ) ;
#36554=CIRCLE ( 'NONE', #68331, 5.000000000000004441 ) ;
#36690=CARTESIAN_POINT ( 'NONE',  ( -48.18343439339133027, -267.2165102598997919, -440.1639404234019253 ) ) ;
#36758=CARTESIAN_POINT ( 'NONE',  ( -43.54160339317392214, -248.0334966641272842, -465.6442049081569508 ) ) ;
#36761=ORIENTED_EDGE ( 'NONE', *, *, #25349, .F. ) ;
#36852=VECTOR ( 'NONE', #42959, 1000.000000000000000 ) ;
#36897=TOROIDAL_SURFACE ( 'NONE', #89789, 204.0731808058633590, 35.00000000000000000 ) ;
#36931=CARTESIAN_POINT ( 'NONE',  ( -48.18343439339133027, -265.6166469183335153, -497.0604155083543105 ) ) ;
#37009=CARTESIAN_POINT ( 'NONE',  ( -43.54160339317392214, -248.0334966641272842, -463.3306390303819740 ) ) ;
#37159=CARTESIAN_POINT ( 'NONE',  ( -48.18343439339133027, -256.0722001994441825, -452.3316844814242472 ) ) ;
#37377=CARTESIAN_POINT ( 'NONE',  ( -48.18343439339132317, -256.9144228299669521, -495.6365959160108332 ) ) ;
#37380=DIRECTION ( 'NONE',  ( 1.000000000000000000, 0.000000000000000000, 0.000000000000000000 ) ) ;
#37697=CARTESIAN_POINT ( 'NONE',  ( -43.45424580659107505, -257.5073373634913878, -441.6910188950594147 ) ) ;
#37835=LINE ( 'NONE', #8502, #38521 ) ;
#37852=EDGE_CURVE ( 'NONE', #33307, #34997, #79241, .T. ) ;
#38159=CARTESIAN_POINT ( 'NONE',  ( -43.21050586802018501, -280.7973836945827770, -430.6442049081568939 ) ) ;
#38211=ORIENTED_EDGE ( 'NONE', *, *, #43955, .T. ) ;
#38248=DIRECTION ( 'NONE',  ( 0.000000000000000000, -1.000000000000000000, 0.000000000000000000 ) ) ;
#38521=VECTOR ( 'NONE', #37380, 1000.000000000000000 ) ;
#38638=CARTESIAN_POINT ( 'NONE',  ( -48.18343439339133027, -266.7963633758117794, -440.4292507800087719 ) ) ;
#39083=CARTESIAN_POINT ( 'NONE',  ( -48.18343439339133027, -281.1257490775032579, -435.6442049083771053 ) ) ;
#39102=CARTESIAN_POINT ( 'NONE',  ( -43.18343439339132317, -283.1093320178188151, -507.6442049081570076 ) ) ;
#39179=DIRECTION ( 'NONE',  ( 1.000000000000000000, 0.000000000000000000, -0.000000000000000000 ) ) ;
#39397=EDGE_LOOP ( 'NONE', ( #29074, #61580, #6089, #31975 ) ) ;
#39542=CARTESIAN_POINT ( 'NONE',  ( -43.35412708609305099, -267.5894485949402224, -434.2348519691648221 ) ) ;
#39559=CARTESIAN_POINT ( 'NONE',  ( -43.28560281309416524, -274.0583670422044520, -506.4787804120613828 ) ) ;
#39561=CARTESIAN_POINT ( 'NONE',  ( -48.18343439339133027, -265.6166469183427807, -497.0604155083162823 ) ) ;
#39623=DIRECTION ( 'NONE',  ( 0.000000000000000000, 1.000000000000000000, -0.000000000000000000 ) ) ;
#39636=CIRCLE ( 'NONE', #92576, 35.00000000000002842 ) ;
#39712=CARTESIAN_POINT ( 'NONE',  ( -48.18343439339133738, -248.5908270566111753, -461.0970999203888141 ) ) ;
#39795=( NAMED_UNIT ( * ) PLANE_ANGLE_UNIT ( ) SI_UNIT ( $, .RADIAN. ) );
#39969=EDGE_CURVE ( 'NONE', #46265, #42209, #67064, .T. ) ;
#40003=CARTESIAN_POINT ( 'NONE',  ( -26.41588298435790350, -486.4924983417995463, -465.6442049081569508 ) ) ;
#40040=FACE_OUTER_BOUND ( 'NONE', #67862, .T. ) ;
#40041=CARTESIAN_POINT ( 'NONE',  ( -48.18343439339133027, -253.0206516614774159, -474.6281350925841025 ) ) ;
#40058=ORIENTED_EDGE ( 'NONE', *, *, #83215, .F. ) ;
#40106=CARTESIAN_POINT ( 'NONE',  ( -43.37497677679506580, -265.5639373360739341, -503.0380110733032666 ) ) ;
#40166=VERTEX_POINT ( 'NONE', #51924 ) ;
#40183=CARTESIAN_POINT ( 'NONE',  ( -48.18343439338617884, -250.5775211731748016, -453.4113254038507534 ) ) ;
#40642=CARTESIAN_POINT ( 'NONE',  ( -48.18343439339133027, -254.4585890652104467, -456.4660217814370071 ) ) ;
#40751=DIRECTION ( 'NONE',  ( 1.000000000000000000, 0.000000000000000000, -0.000000000000000000 ) ) ;
#40773=DIRECTION ( 'NONE',  ( 0.000000000000000000, 0.000000000000000000, 1.000000000000000000 ) ) ;
#41023=CARTESIAN_POINT ( 'NONE',  ( -43.54160339317391504, -248.0334966641272842, -474.9578934535559824 ) ) ;
#41066=ADVANCED_FACE ( 'NONE', ( #15126 ), #43989, .F. ) ;
#41101=VERTEX_POINT ( 'NONE', #8475 ) ;
#41107=CARTESIAN_POINT ( 'NONE',  ( -48.18343439339133027, -248.3668650814815066, -463.3519808654870076 ) ) ;
#41442=CARTESIAN_POINT ( 'NONE',  ( -48.18343439339133027, -253.7029054207625052, -479.0169286797143968 ) ) ;
#41807=ORIENTED_EDGE ( 'NONE', *, *, #69089, .F. ) ;
#41915=CARTESIAN_POINT ( 'NONE',  ( -48.18343439339133027, -254.9503577894309387, -483.2618064832606706 ) ) ;
#42150=EDGE_CURVE ( 'NONE', #2981, #30245, #64319, .T. ) ;
#42191=( NAMED_UNIT ( * ) SI_UNIT ( $, .STERADIAN. ) SOLID_ANGLE_UNIT ( ) );
#42209=VERTEX_POINT ( 'NONE', #70464 ) ;
#42527=EDGE_CURVE ( 'NONE', #46265, #40166, #71684, .T. ) ;
#42628=AXIS2_PLACEMENT_3D ( 'NONE', #52357, #32809, #90531 ) ;
#42723=DIRECTION ( 'NONE',  ( -0.000000000000000000, 0.000000000000000000, -1.000000000000000000 ) ) ;
#42782=VERTEX_POINT ( 'NONE', #3844 ) ;
#42863=CARTESIAN_POINT ( 'NONE',  ( -48.18343439339132317, -256.9970711660894267, -450.6082928460614312 ) ) ;
#42959=DIRECTION ( 'NONE',  ( 0.000000000000000000, 1.000000000000000000, -0.000000000000000000 ) ) ;
#43119=CARTESIAN_POINT ( 'NONE',  ( 41.08708295871279859, -296.0521521680024080, -472.6442049081569508 ) ) ;
#43335=CARTESIAN_POINT ( 'NONE',  ( -48.18343439339133738, -275.2947406849379490, -436.6688341897501573 ) ) ;
#43526=EDGE_CURVE ( 'NONE', #47679, #42209, #72901, .T. ) ;
#43608=ORIENTED_EDGE ( 'NONE', *, *, #22861, .F. ) ;
#43636=CARTESIAN_POINT ( 'NONE',  ( -43.52154907986207633, -250.2679838637678529, -453.2970318977559145 ) ) ;
#43784=CARTESIAN_POINT ( 'NONE',  ( -48.18343439339131606, -259.2349860071790317, -447.3766206888182069 ) ) ;
#43955=EDGE_CURVE ( 'NONE', #58102, #20191, #61852, .T. ) ;
#43989=PLANE ( 'NONE',  #20156 ) ;
#44012=CARTESIAN_POINT ( 'NONE',  ( -48.18343439339133027, -257.5766546844819231, -488.5262689091863990 ) ) ;
#44090=CARTESIAN_POINT ( 'NONE',  ( -43.53958171220627804, -248.2610745740583695, -461.0558268132327271 ) ) ;
#44102=ADVANCED_FACE ( 'NONE', ( #69412 ), #19224, .T. ) ;
#44185=AXIS2_PLACEMENT_3D ( 'NONE', #57439, #56024, #92450 ) ;
#44240=AXIS2_PLACEMENT_3D ( 'NONE', #23842, #89613, #22909 ) ;
#44246=CARTESIAN_POINT ( 'NONE',  ( -48.18343439339132317, -274.8200403470298738, -436.8002545823309219 ) ) ;
#44383=DIRECTION ( 'NONE',  ( -0.000000000000000000, -1.000000000000000000, -0.000000000000000000 ) ) ;
#44407=CARTESIAN_POINT ( 'NONE',  ( -26.41588298435790350, -486.4924983417995463, -472.6442049081569508 ) ) ;
#44418=CIRCLE ( 'NONE', #86729, 35.00000000000003553 ) ;
#44459=DIRECTION ( 'NONE',  ( -0.000000000000000000, -0.000000000000000000, -1.000000000000000000 ) ) ;
#44484=CARTESIAN_POINT ( 'NONE',  ( -48.18343439339133027, -253.0058770677770497, -490.0359438847364686 ) ) ;
#44553=ORIENTED_EDGE ( 'NONE', *, *, #39969, .T. ) ;
#44806=CARTESIAN_POINT ( 'NONE',  ( -48.18343439339133027, -261.8354831489689332, -437.9975051613113806 ) ) ;
#44916=FACE_OUTER_BOUND ( 'NONE', #18843, .T. ) ;
#45041=LINE ( 'NONE', #58368, #76025 ) ;
#45256=CARTESIAN_POINT ( 'NONE',  ( -43.34342893628492277, -268.6218111412664484, -433.7479087153366208 ) ) ;
#45316=CARTESIAN_POINT ( 'NONE',  ( -43.18343439339132317, -486.4924983417995463, -435.6442049081568939 ) ) ;
#45466=LINE ( 'NONE', #53051, #74604 ) ;
#45495=CARTESIAN_POINT ( 'NONE',  ( -43.18343439339132317, -283.1093320178187582, -435.6442049081568939 ) ) ;
#45726=CARTESIAN_POINT ( 'NONE',  ( -43.28619158486827700, -274.0006242052569405, -431.8396057366803120 ) ) ;
#45828=PRODUCT_DEFINITION ( 'UNKNOWN', '', #61340, #55170 ) ;
#45847=DIRECTION ( 'NONE',  ( 0.000000000000000000, -0.000000000000000000, 1.000000000000000000 ) ) ;
#45848=DIRECTION ( 'NONE',  ( -1.000000000000000000, 0.000000000000000000, 0.000000000000000000 ) ) ;
#46108=CLOSED_SHELL ( 'NONE', ( #7407, #41066, #31463, #70445, #29564, #85656, #91968, #67860, #81368, #34993, #13470, #44102, #89366, #78399, #74868, #76860, #3072, #46345, #46385 ) ) ;
#46181=DIRECTION ( 'NONE',  ( 1.000000000000000000, 0.000000000000000000, 0.000000000000000000 ) ) ;
#46200=CARTESIAN_POINT ( 'NONE',  ( -43.36966085509969560, -266.0730555875976506, -435.0432476903218344 ) ) ;
#46220=CARTESIAN_POINT ( 'NONE',  ( -43.41710851680167593, -261.3366415040296715, -500.0926372755047851 ) ) ;
#46222=CARTESIAN_POINT ( 'NONE',  ( -48.18343439339131606, -256.8217696174598927, -487.2503612923801484 ) ) ;
#46265=VERTEX_POINT ( 'NONE', #53010 ) ;
#46345=ADVANCED_FACE ( 'NONE', ( #54410 ), #18912, .T. ) ;
#46385=ADVANCED_FACE ( 'NONE', ( #46823 ), #68182, .T. ) ;
#46386=PRODUCT_CONTEXT ( 'NONE', #31747, 'mechanical' ) ;
#46548=FACE_OUTER_BOUND ( 'NONE', #93012, .T. ) ;
#46658=CARTESIAN_POINT ( 'NONE',  ( -48.18343439339133027, -276.7382201398716006, -436.3198488720709634 ) ) ;
#46678=CARTESIAN_POINT ( 'NONE',  ( -48.18343439337080980, -261.9263060112091921, -500.2732637504696527 ) ) ;
#46680=CARTESIAN_POINT ( 'NONE',  ( -48.18343439339133738, -263.2803689379327921, -495.2320347593006886 ) ) ;
#46745=CARTESIAN_POINT ( 'NONE',  ( -43.52944128795684264, -249.3926482227765860, -482.3108334129058790 ) ) ;
#46823=FACE_OUTER_BOUND ( 'NONE', #21989, .T. ) ;
#47000=LINE ( 'NONE', #63487, #68660 ) ;
#47139=CARTESIAN_POINT ( 'NONE',  ( -48.18343439341874301, -255.4808422879580121, -493.8826162444244119 ) ) ;
#47141=CARTESIAN_POINT ( 'NONE',  ( -48.18343439339133738, -253.7029054207300476, -479.0169286797111567 ) ) ;
#47259=CARTESIAN_POINT ( 'NONE',  ( -46.11236658152585477, -296.0521521680024080, -430.6442049081568371 ) ) ;
#47286=DIRECTION ( 'NONE',  ( -0.000000000000000000, -0.000000000000000000, -1.000000000000000000 ) ) ;
#47563=VERTEX_POINT ( 'NONE', #58928 ) ;
#47620=CARTESIAN_POINT ( 'NONE',  ( -48.18343439339132317, -253.0206516614774728, -474.6280563232480745 ) ) ;
#47644=( GEOMETRIC_REPRESENTATION_CONTEXT ( 3 ) GLOBAL_UNCERTAINTY_ASSIGNED_CONTEXT ( ( #69364 ) ) GLOBAL_UNIT_ASSIGNED_CONTEXT ( ( #13813, #28029, #42191 ) ) REPRESENTATION_CONTEXT ( 'NONE', 'WORKASPACE' ) );
#47654=ORIENTED_EDGE ( 'NONE', *, *, #83488, .F. ) ;
#47679=VERTEX_POINT ( 'NONE', #68355 ) ;
#47687=CARTESIAN_POINT ( 'NONE',  ( -43.41716441663519532, -261.3309580482948036, -500.0881477262567500 ) ) ;
#47767=CARTESIAN_POINT ( 'NONE',  ( -43.54160339317392214, -248.0334966641272558, -465.6442049081569508 ) ) ;
#47808=DIRECTION ( 'NONE',  ( 0.000000000000000000, 0.000000000000000000, 1.000000000000000000 ) ) ;
#48081=CARTESIAN_POINT ( 'NONE',  ( -48.18343439338451617, -250.1980903302585091, -483.8542798561345535 ) ) ;
#48138=PRODUCT_DEFINITION_SHAPE ( 'NONE', 'NONE',  #45828 ) ;
#48147=CARTESIAN_POINT ( 'NONE',  ( -43.53450532834227715, -248.8283547351244067, -480.0763058130885383 ) ) ;
#48160=DIRECTION ( 'NONE',  ( -0.000000000000000000, 1.000000000000000000, -0.000000000000000000 ) ) ;
#48231=CARTESIAN_POINT ( 'NONE',  ( -48.18343439339133027, -258.6462052220223882, -448.1683005986033663 ) ) ;
#48330=EDGE_CURVE ( 'NONE', #42209, #10045, #61277, .T. ) ;
#48442=DIRECTION ( 'NONE',  ( 0.000000000000000000, 0.000000000000000000, -1.000000000000000000 ) ) ;
#48570=B_SPLINE_CURVE_WITH_KNOTS ( 'NONE', 3,
 ( #18832, #68082, #17434, #32575, #91231, #11251, #3207, #89840, #40106, #54329, #26397, #76118, #47687, #82739, #69021, #55285, #17892, #90750, #84139, #12180, #25908, #76589, #69478, #33483, #46745, #62387, #19288, #48147, #77051, #41023, #69948 ),
 .UNSPECIFIED., .F., .F.,
 ( 4, 2, 2, 2, 2, 2, 2, 2, 2, 2, 2, 1, 2, 2, 2, 4 ),
 ( 0.000000000000000000, 0.006842119823167555626, 0.01026317973475138201, 0.01368423964633520840, 0.02052635946950286117, 0.02223688942529476048, 0.02394741938108666326, 0.02736847929267014964, 0.03421059911583700791, 0.03592112907162879620, 0.03763165902742058450, 0.04105271893900415414, 0.04447377885058772379, 0.04618430880637957453, 0.04789483876217142527, 0.05473695858533866865 ),
 .UNSPECIFIED. ) ;
#48848=STYLED_ITEM('',(#93738),#28963);
#48865=AXIS2_PLACEMENT_3D ( 'NONE', #79871, #58577, #72767 ) ;
#48920=VECTOR ( 'NONE', #48160, 1000.000000000000000 ) ;
#49021=DIRECTION ( 'NONE',  ( 0.000000000000000000, 0.000000000000000000, 1.000000000000000000 ) ) ;
#49071=ORIENTED_EDGE ( 'NONE', *, *, #73107, .T. ) ;
#49401=DIRECTION ( 'NONE',  ( 0.000000000000000000, -1.000000000000000000, 0.000000000000000000 ) ) ;
#49506=CARTESIAN_POINT ( 'NONE',  ( -43.50149443762219903, -252.4652299798295019, -489.6847206897468823 ) ) ;
#49759=EDGE_CURVE ( 'NONE', #41101, #86528, #77050, .T. ) ;
#49838=DIRECTION ( 'NONE',  ( 0.000000000000000000, 0.000000000000000000, 1.000000000000000000 ) ) ;
#50359=ORIENTED_EDGE ( 'NONE', *, *, #65811, .T. ) ;
#50361=AXIS2_PLACEMENT_3D ( 'NONE', #29313, #50622, #93689 ) ;
#50414=CIRCLE ( 'NONE', #27718, 35.00000000000000000 ) ;
#50439=CARTESIAN_POINT ( 'NONE',  ( -48.18343439339133738, -268.4940904799720442, -439.4148130071538958 ) ) ;
#50514=ORIENTED_EDGE ( 'NONE', *, *, #65811, .F. ) ;
#50609=EDGE_CURVE ( 'NONE', #47563, #64125, #58833, .T. ) ;
#50622=DIRECTION ( 'NONE',  ( 0.000000000000000000, 0.000000000000000000, 1.000000000000000000 ) ) ;
#50692=DIRECTION ( 'NONE',  ( 0.000000000000000000, 0.000000000000000000, 1.000000000000000000 ) ) ;
#50833=ORIENTED_EDGE ( 'NONE', *, *, #7831, .F. ) ;
#50876=CARTESIAN_POINT ( 'NONE',  ( 41.08708295871279859, -293.9068999365417199, -465.6442049081569508 ) ) ;
#51129=CARTESIAN_POINT ( 'NONE',  ( -48.18343439339133027, -262.5501068226379289, -494.5729214566428027 ) ) ;
#51204=CARTESIAN_POINT ( 'NONE',  ( -43.26782269566163563, -275.6797743861646381, -431.4331960659528704 ) ) ;
#51232=DIRECTION ( 'NONE',  ( -0.000000000000000000, -1.000000000000000000, 0.000000000000000000 ) ) ;
#51410=VERTEX_POINT ( 'NONE', #25617 ) ;
#51578=CARTESIAN_POINT ( 'NONE',  ( -48.18343439339133027, -257.0657538259594617, -487.6787901984638438 ) ) ;
#51924=CARTESIAN_POINT ( 'NONE',  ( 41.08708295871279859, -293.9068999365417199, -507.6442049081570076 ) ) ;
#51987=AXIS2_PLACEMENT_3D ( 'NONE', #64364, #93190, #35902 ) ;
#52012=ORIENTED_EDGE ( 'NONE', *, *, #36276, .T. ) ;
#52026=CIRCLE ( 'NONE', #5211, 35.00000000000000000 ) ;
#52057=CARTESIAN_POINT ( 'NONE',  ( -43.43851610984211220, -259.1436342284649186, -498.2277075480836288 ) ) ;
#52058=AXIS2_PLACEMENT_3D ( 'NONE', #70156, #77718, #40751 ) ;
#52357=CARTESIAN_POINT ( 'NONE',  ( 76.08708295871279859, -296.0521521680024080, -430.6442049081568939 ) ) ;
#52807=DIRECTION ( 'NONE',  ( -0.000000000000000000, 0.000000000000000000, -1.000000000000000000 ) ) ;
#52841=CARTESIAN_POINT ( 'NONE',  ( -48.18343439341505530, -270.7767787986900316, -433.0017230881019827 ) ) ;
#52861=CARTESIAN_POINT ( 'NONE',  ( -48.18343439339133027, -253.2160367275913018, -476.5905725147042062 ) ) ;
#52977=AXIS2_PLACEMENT_3D ( 'NONE', #25732, #49401, #48442 ) ;
#53010=CARTESIAN_POINT ( 'NONE',  ( -43.18343439339132317, -283.1093320178187582, -507.6442049081570076 ) ) ;
#53051=CARTESIAN_POINT ( 'NONE',  ( -48.18343439339133027, -253.0206516614774728, -430.6442049081568939 ) ) ;
#53310=CARTESIAN_POINT ( 'NONE',  ( -48.18343439339478351, -271.8438693890086029, -432.6084584992419195 ) ) ;
#53649=ORIENTED_EDGE ( 'NONE', *, *, #28009, .T. ) ;
#53788=CARTESIAN_POINT ( 'NONE',  ( -43.38969887572877582, -264.0939091915531662, -436.2267584252900292 ) ) ;
#53808=CARTESIAN_POINT ( 'NONE',  ( -48.18343439336388201, -280.8035638491393229, -507.6172057986060508 ) ) ;
#53952=CARTESIAN_POINT ( 'NONE',  ( -48.18343439338273981, -255.8486676696398376, -444.0454921972241209 ) ) ;
#54092=ORIENTED_EDGE ( 'NONE', *, *, #32585, .T. ) ;
#54245=CARTESIAN_POINT ( 'NONE',  ( -48.18343439337095191, -257.6947538200772101, -441.8664075291517861 ) ) ;
#54262=CARTESIAN_POINT ( 'NONE',  ( -48.18343439339133027, -259.2200010660633893, -490.9919136895239262 ) ) ;
#54264=CARTESIAN_POINT ( 'NONE',  ( -48.18343439339133027, -273.4572633954001049, -501.0766502680399412 ) ) ;
#54329=CARTESIAN_POINT ( 'NONE',  ( -43.39882518443393167, -263.1823801016103630, -501.4546314904750943 ) ) ;
#54380=CARTESIAN_POINT ( 'NONE',  ( -48.18343439339133027, -293.9810843561368756, -432.7152727200224263 ) ) ;
#54410=FACE_OUTER_BOUND ( 'NONE', #60128, .T. ) ;
#54723=CARTESIAN_POINT ( 'NONE',  ( -48.18343439339474088, -249.7038996752085040, -482.2249225752359507 ) ) ;
#54786=DIRECTION ( 'NONE',  ( 0.000000000000000000, 0.000000000000000000, 1.000000000000000000 ) ) ;
#54876=CARTESIAN_POINT ( 'NONE',  ( -43.53958015783998547, -248.2612498862057180, -461.0541023492486943 ) ) ;
#55085=CARTESIAN_POINT ( 'NONE',  ( -48.18343439339133027, -248.4123448508205172, -502.6442049081569508 ) ) ;
#55166=AXIS2_PLACEMENT_3D ( 'NONE', #22707, #1867, #22260 ) ;
#55170=PRODUCT_DEFINITION_CONTEXT ( 'detailed design', #57215, 'design' ) ;
#55219=CARTESIAN_POINT ( 'NONE',  ( -43.54160339317392214, -248.0334966641273127, -472.6442049081569508 ) ) ;
#55285=CARTESIAN_POINT ( 'NONE',  ( -43.46191054614098448, -256.7101074799442131, -495.8041560030679307 ) ) ;
#55367=CARTESIAN_POINT ( 'NONE',  ( -43.49966619312522909, -252.6696169169302948, -448.1023075023964566 ) ) ;
#55684=CARTESIAN_POINT ( 'NONE',  ( -48.18343439339133027, -254.1872365014273782, -480.9328361744520066 ) ) ;
#55829=CARTESIAN_POINT ( 'NONE',  ( -48.18343439339133027, -259.5409938267127359, -446.9856792133372778 ) ) ;
#55877=DIRECTION ( 'NONE',  ( 1.000000000000000000, 0.000000000000000000, 0.000000000000000000 ) ) ;
#56024=DIRECTION ( 'NONE',  ( 0.000000000000000000, 0.000000000000000000, 1.000000000000000000 ) ) ;
#56044=CARTESIAN_POINT ( 'NONE',  ( -48.18343439339133027, -291.0521521680024080, -502.6442049081569508 ) ) ;
#56151=CARTESIAN_POINT ( 'NONE',  ( -48.18343439339133027, -253.2160367274611872, -476.5905725146912459 ) ) ;
#56209=ORIENTED_EDGE ( 'NONE', *, *, #49759, .F. ) ;
#56504=FACE_OUTER_BOUND ( 'NONE', #39397, .T. ) ;
#56639=CARTESIAN_POINT ( 'NONE',  ( -48.18343439340156209, -251.9247748416627530, -488.0338856575309592 ) ) ;
#57101=CARTESIAN_POINT ( 'NONE',  ( -48.18343439339133738, -260.4846106489495128, -445.8398854946861434 ) ) ;
#57215=APPLICATION_CONTEXT ( 'automotive_design' ) ;
#57439=CARTESIAN_POINT ( 'NONE',  ( -26.41588298435790350, -486.4924983417995463, -430.6442049081568939 ) ) ;
#57711=FACE_OUTER_BOUND ( 'NONE', #17636, .T. ) ;
#57864=CARTESIAN_POINT ( 'NONE',  ( -43.41372958812449667, -261.6932476095567495, -437.8285871551558444 ) ) ;
#58102=VERTEX_POINT ( 'NONE', #16758 ) ;
#58159=VERTEX_POINT ( 'NONE', #81609 ) ;
#58303=ORIENTED_EDGE ( 'NONE', *, *, #66289, .F. ) ;
#58342=CARTESIAN_POINT ( 'NONE',  ( -43.30994550414099109, -271.7986277240285062, -432.4934747601029699 ) ) ;
#58368=CARTESIAN_POINT ( 'NONE',  ( 41.08708295871279859, -486.4924983417995463, -507.6442049081570076 ) ) ;
#58577=DIRECTION ( 'NONE',  ( 0.000000000000000000, 1.000000000000000000, -0.000000000000000000 ) ) ;
#58714=CARTESIAN_POINT ( 'NONE',  ( -48.18343439338448775, -253.8987417476172368, -491.5047106340448977 ) ) ;
#58833=LINE ( 'NONE', #81057, #87569 ) ;
#58928=CARTESIAN_POINT ( 'NONE',  ( 76.08708295871279859, -293.9068999365417199, -465.6442049081569508 ) ) ;
#58946=CARTESIAN_POINT ( 'NONE',  ( -48.18343439339132317, -264.7419918502895371, -441.7985027590103186 ) ) ;
#59174=CARTESIAN_POINT ( 'NONE',  ( -48.18343439339471956, -275.1886040666647659, -506.6685929469949201 ) ) ;
#59255=CARTESIAN_POINT ( 'NONE',  ( -43.46163685640959784, -256.7309459520654968, -442.5444711093502406 ) ) ;
#59476=EDGE_CURVE ( 'NONE', #20191, #33307, #4302, .T. ) ;
#59514=CARTESIAN_POINT ( 'NONE',  ( -48.18343439306194398, -280.8036219927305410, -430.6712033366062542 ) ) ;
#59999=CARTESIAN_POINT ( 'NONE',  ( -48.18343439339133738, -279.1747503396557590, -502.4506777725324014 ) ) ;
#60128=EDGE_LOOP ( 'NONE', ( #33147, #60737, #25194, #41807 ) ) ;
#60441=CARTESIAN_POINT ( 'NONE',  ( -48.18343439343216517, -260.0909709188723014, -439.4475977827055999 ) ) ;
#60461=CARTESIAN_POINT ( 'NONE',  ( -48.18343439339134449, -281.1255779508778119, -502.6442049081570644 ) ) ;
#60679=DIRECTION ( 'NONE',  ( 0.000000000000000000, 0.000000000000000000, 1.000000000000000000 ) ) ;
#60737=ORIENTED_EDGE ( 'NONE', *, *, #64244, .F. ) ;
#60903=CARTESIAN_POINT ( 'NONE',  ( -43.41367318021437427, -261.6989687524993542, -437.8242190674686753 ) ) ;
#60922=CARTESIAN_POINT ( 'NONE',  ( -43.37491821897447153, -265.5697000172091293, -503.0412998836937390 ) ) ;
#60995=AXIS2_PLACEMENT_3D ( 'NONE', #8831, #8379, #9290 ) ;
#61150=LINE ( 'NONE', #2893, #35291 ) ;
#61277=LINE ( 'NONE', #55085, #16486 ) ;
#61340=PRODUCT_DEFINITION_FORMATION_WITH_SPECIFIED_SOURCE ( 'ANY', '', #28567, .NOT_KNOWN. ) ;
#61383=CARTESIAN_POINT ( 'NONE',  ( -48.18343439336755551, -268.6864615527640012, -433.8888687766993826 ) ) ;
#61401=CARTESIAN_POINT ( 'NONE',  ( -43.46186634799974513, -256.7147672836524066, -495.8094554426511991 ) ) ;
#61403=CARTESIAN_POINT ( 'NONE',  ( -48.18343439339132317, -266.0193969580586781, -497.3422536412688828 ) ) ;
#61580=ORIENTED_EDGE ( 'NONE', *, *, #91011, .F. ) ;
#61799=EDGE_CURVE ( 'NONE', #86528, #58102, #22202, .T. ) ;
#61851=CARTESIAN_POINT ( 'NONE',  ( -48.18343439339133027, -273.4572633953990248, -501.0766502679427958 ) ) ;
#61852=LINE ( 'NONE', #25843, #13333 ) ;
#61995=CARTESIAN_POINT ( 'NONE',  ( -48.18343439339135159, -251.8661507411202365, -450.2476286390481164 ) ) ;
#62145=EDGE_CURVE ( 'NONE', #46265, #51410, #48570, .T. ) ;
#62240=ORIENTED_EDGE ( 'NONE', *, *, #62639, .T. ) ;
#62319=CARTESIAN_POINT ( 'NONE',  ( -48.18343439339133027, -256.8217696174888829, -487.2503612923645733 ) ) ;
#62387=CARTESIAN_POINT ( 'NONE',  ( -43.53082812742030683, -249.2383276863598383, -481.7579445234451327 ) ) ;
#62403=LINE ( 'NONE', #91721, #48920 ) ;
#62475=CARTESIAN_POINT ( 'NONE',  ( -48.18343439339133027, -253.7899642232936515, -458.8318842538573676 ) ) ;
#62608=EDGE_LOOP ( 'NONE', ( #43608, #17052, #8460, #68301 ) ) ;
#62639=EDGE_CURVE ( 'NONE', #10045, #87518, #6024, .T. ) ;
#62956=CARTESIAN_POINT ( 'NONE',  ( -48.18343439339819412, -255.4970356414862067, -444.4998647227852757 ) ) ;
#63166=EDGE_LOOP ( 'NONE', ( #12629, #16846, #15204, #22185, #75421, #81121 ) ) ;
#63277=CARTESIAN_POINT ( 'NONE',  ( -48.18343439339133027, -254.6182378140498486, -482.3412084739298962 ) ) ;
#63487=CARTESIAN_POINT ( 'NONE',  ( -43.54160339317392214, -248.0334966641272842, -430.6442049081568939 ) ) ;
#63703=ORIENTED_EDGE ( 'NONE', *, *, #27878, .F. ) ;
#64125=VERTEX_POINT ( 'NONE', #16611 ) ;
#64130=VECTOR ( 'NONE', #19727, 1000.000000000000000 ) ;
#64244=EDGE_CURVE ( 'NONE', #42782, #47679, #45466, .T. ) ;
#64299=CARTESIAN_POINT ( 'NONE',  ( -43.18343439339132317, -253.0206516614774159, -472.6442049081569508 ) ) ;
#64319=LINE ( 'NONE', #13624, #36852 ) ;
#64364=CARTESIAN_POINT ( 'NONE',  ( -26.41588298435790350, -486.4924983417995463, -465.6442049081569508 ) ) ;
#64506=SHAPE_REPRESENTATION_RELATIONSHIP ( 'NONE' , 'NONE' ,  #30030, #2316 ) ;
#64540=CARTESIAN_POINT ( 'NONE',  ( -43.28623554199135270, -273.9965794730779862, -431.8406871970819907 ) ) ;
#64655=EDGE_CURVE ( 'NONE', #30245, #58159, #50414, .T. ) ;
#64884=EDGE_CURVE ( 'NONE', #58159, #51410, #33785, .T. ) ;
#64997=CARTESIAN_POINT ( 'NONE',  ( -43.49969339204867680, -252.6666589713051394, -448.1074777562126314 ) ) ;
#65146=CARTESIAN_POINT ( 'NONE',  ( -48.18343439339133027, -283.1093320178187582, -435.6442049081568939 ) ) ;
#65738=( BOUNDED_CURVE ( )  B_SPLINE_CURVE ( 3, ( #69278, #3953, #26661, #10566 ),
 .UNSPECIFIED., .F., .F. ) 
 B_SPLINE_CURVE_WITH_KNOTS ( ( 4, 4 ),
 ( 4.712388980384689674, 6.283185307179586232 ),
 .UNSPECIFIED. ) 
 CURVE ( )  GEOMETRIC_REPRESENTATION_ITEM ( )  RATIONAL_B_SPLINE_CURVE ( ( 1.000000000000000000, 0.8047378541243649375, 0.8047378541243649375, 1.000000000000000000 ) ) 
 REPRESENTATION_ITEM ( '' )  );
#65811=EDGE_CURVE ( 'NONE', #89245, #46265, #86594, .T. ) ;
#65845=CARTESIAN_POINT ( 'NONE',  ( -48.18343439339133027, -274.0850372458094171, -506.3822550525310362 ) ) ;
#65922=CARTESIAN_POINT ( 'NONE',  ( -43.45429243013615661, -257.5024557858946537, -441.6962169675167047 ) ) ;
#66068=CARTESIAN_POINT ( 'NONE',  ( -48.18343439339131606, -254.9385145489663103, -455.0573192304916006 ) ) ;
#66287=CARTESIAN_POINT ( 'NONE',  ( -43.49887528382338786, -252.7496869255646459, -490.1845544134979491 ) ) ;
#66289=EDGE_CURVE ( 'NONE', #87518, #41101, #62403, .T. ) ;
#66402=DIRECTION ( 'NONE',  ( 0.000000000000000000, -1.000000000000000000, 0.000000000000000000 ) ) ;
#66434=EDGE_LOOP ( 'NONE', ( #40058, #54092, #63703, #88552 ) ) ;
#66603=CARTESIAN_POINT ( 'NONE',  ( -48.18343439339133027, -264.7419918502239398, -441.7985027589016909 ) ) ;
#66667=ORIENTED_EDGE ( 'NONE', *, *, #67205, .T. ) ;
#66751=EDGE_LOOP ( 'NONE', ( #28911, #12974, #53649 ) ) ;
#66830=VECTOR ( 'NONE', #25148, 1000.000000000000000 ) ;
#66890=ORIENTED_EDGE ( 'NONE', *, *, #83986, .T. ) ;
#67064=CIRCLE ( 'NONE', #60995, 5.000000000000004441 ) ;
#67095=CARTESIAN_POINT ( 'NONE',  ( -48.18343439339132317, -264.4312075782299303, -496.1714326515946709 ) ) ;
#67175=ORIENTED_EDGE ( 'NONE', *, *, #32585, .F. ) ;
#67192=CARTESIAN_POINT ( 'NONE',  ( -26.41588298435790350, -486.4924983417995463, -430.6442049081568939 ) ) ;
#67205=EDGE_CURVE ( 'NONE', #30245, #47563, #80785, .T. ) ;
#67321=DIRECTION ( 'NONE',  ( 0.000000000000000000, 1.000000000000000000, -0.000000000000000000 ) ) ;
#67541=CARTESIAN_POINT ( 'NONE',  ( -48.18343439339133027, -270.6804750412892986, -438.3045224571701510 ) ) ;
#67860=ADVANCED_FACE ( 'NONE', ( #82638 ), #36897, .T. ) ;
#67862=EDGE_LOOP ( 'NONE', ( #44553, #11540, #33262, #13582 ) ) ;
#67997=CARTESIAN_POINT ( 'NONE',  ( -48.18343439339133027, -283.1093320178187582, -435.6442049081568939 ) ) ;
#68014=CARTESIAN_POINT ( 'NONE',  ( -43.30930410892831617, -271.8587292610232566, -505.8153911613401306 ) ) ;
#68082=CARTESIAN_POINT ( 'NONE',  ( -43.21052260110369758, -280.7959546627067766, -507.6442049081571213 ) ) ;
#68182=( BOUNDED_SURFACE ( )  B_SPLINE_SURFACE ( 3, 2, ( 
 ( #4229, #11792, #47767 ),
 ( #26941, #41107, #33106 ),
 ( #26478, #39712, #54876 ),
 ( #62475, #10848, #75726 ),
 ( #77133, #76665, #3769 ),
 ( #40642, #90831, #12264 ),
 ( #91317, #32654, #69562 ),
 ( #82819, #40183, #70038 ),
 ( #25990, #4690, #90375 ),
 ( #18427, #61995, #19366 ),
 ( #33565, #25530, #55367 ),
 ( #84219, #76203, #11332 ),
 ( #48231, #34054, #69102 ),
 ( #5179, #62956, #91790 ),
 ( #55829, #53952, #83115 ),
 ( #88819, #25365, #75105 ),
 ( #74636, #54245, #37697 ),
 ( #32005, #60441, #9763 ),
 ( #66603, #44806, #60903 ),
 ( #38638, #89751, #53788 ),
 ( #81259, #31549, #23967 ),
 ( #73707, #24911, #82195 ),
 ( #74160, #2208, #46200 ),
 ( #9276, #10684, #39542 ),
 ( #67541, #61383, #45256 ),
 ( #3125, #52841, #89277 ),
 ( #10215, #53310, #1725 ),
 ( #81718, #90216, #16867 ),
 ( #16404, #8817, #45726 ),
 ( #82656, #2670, #24428 ),
 ( #46658, #75562, #17349 ),
 ( #17805, #68464, #30612 ),
 ( #39083, #59514, #38159 ),
 ( #67997, #3599, #32486 ) ),
 .UNSPECIFIED., .F., .F., .F. ) 
 B_SPLINE_SURFACE_WITH_KNOTS ( ( 4, 2, 2, 2, 2, 2, 2, 2, 2, 2, 2, 2, 2, 2, 2, 2, 4 ),
 ( 3, 3 ),
 ( 0.000000000000000000, 0.005866933686059443154, 0.008800400529089164731, 0.01026713395060402552, 0.01173386737211888631, 0.01760080105817832946, 0.01906753447969319198, 0.02053426790120805104, 0.02346773474423777261, 0.02933466843029721577, 0.03080140185181207482, 0.03226813527332693388, 0.03520160211635665892, 0.03813506895938638397, 0.03960180238090124649, 0.04106853580241610208, 0.04693546948847554523 ),
 ( 0.000000000000000000, 1.000000000000000000 ),
 .UNSPECIFIED. ) 
 GEOMETRIC_REPRESENTATION_ITEM ( )  RATIONAL_B_SPLINE_SURFACE ( (
 ( 1.000000000000000000, 0.7319951502423088785, 1.000000000000000000),
 ( 1.000000000000000000, 0.7319945071636718703, 1.000000000000000000),
 ( 1.000000000000000000, 0.7318569880056964294, 1.000000000000000000),
 ( 1.000000000000000000, 0.7314477122716916968, 1.000000000000000000),
 ( 1.000000000000000000, 0.7312773020566604165, 1.000000000000000000),
 ( 1.000000000000000000, 0.7309684991269558285, 1.000000000000000000),
 ( 1.000000000000000000, 0.7308564438270946928, 1.000000000000000000),
 ( 1.000000000000000000, 0.7306150055450980618, 1.000000000000000000),
 ( 1.000000000000000000, 0.7304861486422284944, 1.000000000000000000),
 ( 1.000000000000000000, 0.7298013683911470650, 1.000000000000000000),
 ( 1.000000000000000000, 0.7291253948077436320, 1.000000000000000000),
 ( 1.000000000000000000, 0.7281088291350222841, 1.000000000000000000),
 ( 1.000000000000000000, 0.7278968450267667700, 1.000000000000000000),
 ( 1.000000000000000000, 0.7274548661943022188, 1.000000000000000000),
 ( 1.000000000000000000, 0.7272241993259396242, 1.000000000000000000),
 ( 1.000000000000000000, 0.7265094949468547947, 1.000000000000000000),
 ( 1.000000000000000000, 0.7260037385991419123, 1.000000000000000000),
 ( 1.000000000000000000, 0.7243961799752839381, 1.000000000000000000),
 ( 1.000000000000000000, 0.7232051185136439964, 1.000000000000000000),
 ( 1.000000000000000000, 0.7215445644803780700, 1.000000000000000000),
 ( 1.000000000000000000, 0.7212028694993208866, 1.000000000000000000),
 ( 1.000000000000000000, 0.7205081462822442440, 1.000000000000000000),
 ( 1.000000000000000000, 0.7201546886187416563, 1.000000000000000000),
 ( 1.000000000000000000, 0.7190756474479115257, 1.000000000000000000),
 ( 1.000000000000000000, 0.7183314332535508662, 1.000000000000000000),
 ( 1.000000000000000000, 0.7167903837648086363, 1.000000000000000000),
 ( 1.000000000000000000, 0.7159935541304642825, 1.000000000000000000),
 ( 1.000000000000000000, 0.7147557110474020980, 1.000000000000000000),
 ( 1.000000000000000000, 0.7143359865066217784, 1.000000000000000000),
 ( 1.000000000000000000, 0.7134816549837853517, 1.000000000000000000),
 ( 1.000000000000000000, 0.7130464429203826615, 1.000000000000000000),
 ( 1.000000000000000000, 0.7108513879084432663, 1.000000000000000000),
 ( 1.000000000000000000, 0.7090209741736491766, 1.000000000000000000),
 ( 1.000000000000000000, 0.7071067811865441310, 1.000000000000000000) ) ) 
 REPRESENTATION_ITEM ( '' )  SURFACE ( )  );
#68301=ORIENTED_EDGE ( 'NONE', *, *, #59476, .F. ) ;
#68331=AXIS2_PLACEMENT_3D ( 'NONE', #64299, #6500, #71846 ) ;
#68355=CARTESIAN_POINT ( 'NONE',  ( -48.18343439339133027, -253.0206516614774728, -472.6442049081569508 ) ) ;
#68394=VECTOR ( 'NONE', #38248, 1000.000000000000000 ) ;
#68464=CARTESIAN_POINT ( 'NONE',  ( -48.18343439343948376, -278.5213373408708435, -430.9214249866280397 ) ) ;
#68481=CARTESIAN_POINT ( 'NONE',  ( -43.41260863027326877, -261.7933826436608342, -500.4472285273179182 ) ) ;
#68483=CARTESIAN_POINT ( 'NONE',  ( -48.18343439339133027, -254.6182378140904916, -482.3412084739035208 ) ) ;
#68515=ORIENTED_EDGE ( 'NONE', *, *, #64655, .T. ) ;
#68628=CIRCLE ( 'NONE', #51987, 239.0731808058633590 ) ;
#68636=CARTESIAN_POINT ( 'NONE',  ( -43.18343439339132317, -253.0206516614774728, -430.6442049081568939 ) ) ;
#68660=VECTOR ( 'NONE', #10561, 1000.000000000000000 ) ;
#68911=B_SPLINE_CURVE_WITH_KNOTS ( 'NONE', 3,
 ( #80092, #37009, #44090, #7204, #1481, #36079, #43636, #35625, #64997, #100, #15234, #78706, #28979, #59255, #65922, #20941, #57864, #86720, #72534, #13848, #7653, #28516, #29454, #58342, #87184, #64540, #93366, #51204, #72994, #1034, #87640 ),
 .UNSPECIFIED., .F., .F.,
 ( 4, 2, 2, 2, 2, 2, 2, 2, 2, 2, 2, 1, 2, 2, 2, 4 ),
 ( 0.000000000000000000, 0.006842209725270028201, 0.01026331458790513164, 0.01368441945054023508, 0.02052662917581044369, 0.02223718160712799194, 0.02394773403844554713, 0.02736883890108088302, 0.03421104862635143684, 0.03592160105766905448, 0.03763215348898667212, 0.04105325835162196985, 0.04447436321425726757, 0.04618491564557489909, 0.04789546807689253061, 0.05473767780216309137 ),
 .UNSPECIFIED. ) ;
#68922=EDGE_CURVE ( 'NONE', #47563, #34997, #52026, .T. ) ;
#68956=CARTESIAN_POINT ( 'NONE',  ( -48.18343439339133027, -279.1747503396363186, -502.4506777725899838 ) ) ;
#69021=CARTESIAN_POINT ( 'NONE',  ( -43.43856716719556488, -259.1383543305317971, -498.2227791763972391 ) ) ;
#69089=EDGE_CURVE ( 'NONE', #51410, #30930, #47000, .T. ) ;
#69102=CARTESIAN_POINT ( 'NONE',  ( -43.48177207501702668, -254.5922926149944487, -445.2556498803733120 ) ) ;
#69278=CARTESIAN_POINT ( 'NONE',  ( -48.18343439339133027, -291.0521521680024080, -502.6442049081569508 ) ) ;
#69364=UNCERTAINTY_MEASURE_WITH_UNIT (LENGTH_MEASURE( 1.000000000000000082E-05 ), #13813, 'distance_accuracy_value', 'NONE');
#69411=CARTESIAN_POINT ( 'NONE',  ( -48.18343439339304268, -249.1487204936213971, -480.0094059802160018 ) ) ;
#69412=FACE_OUTER_BOUND ( 'NONE', #62608, .T. ) ;
#69478=CARTESIAN_POINT ( 'NONE',  ( -43.51792863845375336, -250.6687662136113488, -486.1009916026080759 ) ) ;
#69562=CARTESIAN_POINT ( 'NONE',  ( -43.52494566250408070, -249.8916412613903901, -454.3875622718719569 ) ) ;
#69916=ORIENTED_EDGE ( 'NONE', *, *, #48330, .T. ) ;
#69948=CARTESIAN_POINT ( 'NONE',  ( -43.54160339317392214, -248.0334966641272842, -472.6442049081569508 ) ) ;
#70038=CARTESIAN_POINT ( 'NONE',  ( -43.52141711092885146, -250.2819871534461242, -453.2997318089873033 ) ) ;
#70156=CARTESIAN_POINT ( 'NONE',  ( -26.41588298435790350, -486.4924983417995463, -507.6442049081570076 ) ) ;
#70181=AXIS2_PLACEMENT_3D ( 'NONE', #45316, #74220, #9339 ) ;
#70374=CARTESIAN_POINT ( 'NONE',  ( -48.18343439339133027, -248.3668650810961083, -474.9365983928495893 ) ) ;
#70445=ADVANCED_FACE ( 'NONE', ( #44916 ), #74272, .T. ) ;
#70464=CARTESIAN_POINT ( 'NONE',  ( -48.18343439339133027, -283.1093320178187582, -502.6442049081569508 ) ) ;
#70721=FACE_OUTER_BOUND ( 'NONE', #15920, .T. ) ;
#70828=CARTESIAN_POINT ( 'NONE',  ( -48.18343439339133027, -254.0547856900534214, -480.4587914081801614 ) ) ;
#71045=CYLINDRICAL_SURFACE ( 'NONE', #26284, 35.00000000000000000 ) ;
#71168=DIRECTION ( 'NONE',  ( -1.000000000000000000, 0.000000000000000000, 0.000000000000000000 ) ) ;
#71684=CIRCLE ( 'NONE', #88266, 204.0731808058633590 ) ;
#71777=CARTESIAN_POINT ( 'NONE',  ( -48.18343439339134449, -258.6462052220593932, -448.1683005986229205 ) ) ;
#71805=( BOUNDED_SURFACE ( )  B_SPLINE_SURFACE ( 3, 2, ( 
 ( #1400, #10234, #39102 ),
 ( #80940, #53808, #80464 ),
 ( #68956, #30287, #89769 ),
 ( #4087, #59174, #76049 ),
 ( #90233, #65845, #39559 ),
 ( #61851, #75124, #68014 ),
 ( #88019, #82676, #3143 ),
 ( #17825, #32958, #83132 ),
 ( #8499, #32025, #60922 ),
 ( #18283, #75581, #8036 ),
 ( #36931, #24931, #29831 ),
 ( #72910, #46678, #68481 ),
 ( #3617, #25382, #46220 ),
 ( #22256, #23175, #15613 ),
 ( #51129, #73389, #52057 ),
 ( #32504, #37377, #61401 ),
 ( #54262, #47139, #953 ),
 ( #11180, #58714, #80012 ),
 ( #44012, #87558, #22704 ),
 ( #51578, #44484, #66287 ),
 ( #62319, #20636, #49506 ),
 ( #83599, #56639, #34372 ),
 ( #33902, #5021, #25842 ),
 ( #41915, #26798, #84073 ),
 ( #63277, #48081, #76523 ),
 ( #55684, #54723, #92110 ),
 ( #70828, #27264, #19682 ),
 ( #18762, #4542, #91644 ),
 ( #41442, #69411, #12115 ),
 ( #56151, #13079, #34834 ),
 ( #47620, #70374, #5499 ),
 ( #84535, #85006, #55219 ) ),
 .UNSPECIFIED., .F., .F., .F. ) 
 B_SPLINE_SURFACE_WITH_KNOTS ( ( 4, 2, 2, 2, 2, 2, 2, 2, 2, 2, 2, 2, 2, 2, 2, 4 ),
 ( 3, 3 ),
 ( 0.000000000000000000, 0.005866952128964776289, 0.008800428193447163566, 0.01173390425792955258, 0.01760085638689432713, 0.01906759441913552164, 0.02053433245137671614, 0.02346780851585910516, 0.02933476064482387971, 0.03080149867706507422, 0.03226823670930626525, 0.03520171277378865426, 0.03813518883827104328, 0.03960192687051224125, 0.04106866490275343229, 0.04693561703171821031 ),
 ( 0.000000000000000000, 1.000000000000000000 ),
 .UNSPECIFIED. ) 
 GEOMETRIC_REPRESENTATION_ITEM ( )  RATIONAL_B_SPLINE_SURFACE ( (
 ( 1.000000000000000000, 0.7071067811865480168, 1.000000000000000000),
 ( 1.000000000000000000, 0.7090210024396556010, 1.000000000000000000),
 ( 1.000000000000000000, 0.7108407973597864471, 1.000000000000000000),
 ( 1.000000000000000000, 0.7134470143025161137, 1.000000000000000000),
 ( 1.000000000000000000, 0.7142951270337911662, 1.000000000000000000),
 ( 1.000000000000000000, 0.7159522736098768991, 1.000000000000000000),
 ( 1.000000000000000000, 0.7167636429391108788, 1.000000000000000000),
 ( 1.000000000000000000, 0.7190918835810566900, 1.000000000000000000),
 ( 1.000000000000000000, 0.7205207347168143261, 1.000000000000000000),
 ( 1.000000000000000000, 0.7221727232895018833, 1.000000000000000000),
 ( 1.000000000000000000, 0.7224963568879022580, 1.000000000000000000),
 ( 1.000000000000000000, 0.7231303645827314996, 1.000000000000000000),
 ( 1.000000000000000000, 0.7234414309858798742, 1.000000000000000000),
 ( 1.000000000000000000, 0.7243500205383740509, 1.000000000000000000),
 ( 1.000000000000000000, 0.7249196227328268405, 1.000000000000000000),
 ( 1.000000000000000000, 0.7265289715998781706, 1.000000000000000000),
 ( 1.000000000000000000, 0.7274702368494421201, 1.000000000000000000),
 ( 1.000000000000000000, 0.7284953164274693416, 1.000000000000000000),
 ( 1.000000000000000000, 0.7286931934763172247, 1.000000000000000000),
 ( 1.000000000000000000, 0.7290707267997620367, 1.000000000000000000),
 ( 1.000000000000000000, 0.7292503229930066277, 1.000000000000000000),
 ( 1.000000000000000000, 0.7297626290626116896, 1.000000000000000000),
 ( 1.000000000000000000, 0.7300689337816327340, 1.000000000000000000),
 ( 1.000000000000000000, 0.7306145467741796962, 1.000000000000000000),
 ( 1.000000000000000000, 0.7308538497138195034, 1.000000000000000000),
 ( 1.000000000000000000, 0.7311633277236124773, 1.000000000000000000),
 ( 1.000000000000000000, 0.7312582226261189478, 1.000000000000000000),
 ( 1.000000000000000000, 0.7314313872177583553, 1.000000000000000000),
 ( 1.000000000000000000, 0.7315097857000790738, 1.000000000000000000),
 ( 1.000000000000000000, 0.7318569749151436765, 1.000000000000000000),
 ( 1.000000000000000000, 0.7319944972810035200, 1.000000000000000000),
 ( 1.000000000000000000, 0.7319951502423088785, 1.000000000000000000) ) ) 
 REPRESENTATION_ITEM ( '' )  SURFACE ( )  );
#71846=DIRECTION ( 'NONE',  ( 1.000000000000000000, 0.000000000000000000, 0.000000000000000000 ) ) ;
#71954=EDGE_LOOP ( 'NONE', ( #31799, #21853, #38211, #83295 ) ) ;
#72534=CARTESIAN_POINT ( 'NONE',  ( -43.38482778162041598, -264.5778734463897877, -435.9208459153147714 ) ) ;
#72754=DIRECTION ( 'NONE',  ( -0.000000000000000000, -0.000000000000000000, 1.000000000000000000 ) ) ;
#72767=DIRECTION ( 'NONE',  ( 0.000000000000000000, 0.000000000000000000, 1.000000000000000000 ) ) ;
#72886=CARTESIAN_POINT ( 'NONE',  ( -48.18343439339133027, -296.0521521680024080, -430.6442049081568939 ) ) ;
#72901=B_SPLINE_CURVE_WITH_KNOTS ( 'NONE', 3,
 ( #89296, #40041, #52861, #47141, #2690, #3619, #24451, #68483, #83134, #23533, #46222, #10236, #81279, #81739, #89771, #31571, #17828, #46680, #67095, #74180, #39561, #61403, #32506, #2229, #75126, #54264, #90235, #31112, #59999, #60461, #25384 ),
 .UNSPECIFIED., .F., .F.,
 ( 4, 2, 2, 2, 1, 2, 2, 2, 2, 2, 2, 2, 2, 2, 2, 4 ),
 ( 0.000000000000000000, 0.005916104402640001356, 0.007395130503299944882, 0.008874156603959888409, 0.01183220880527966271, 0.01479026100659944047, 0.01626928710725932675, 0.01774831320791921477, 0.02366441761055876683, 0.02662246981187848041, 0.02810149591253845516, 0.02958052201319842645, 0.03549662641583841566, 0.03845467861715847618, 0.04141273081847853671, 0.04732883522111848429 ),
 .UNSPECIFIED. ) ;
#72910=CARTESIAN_POINT ( 'NONE',  ( -48.18343439339133027, -264.8229914578195121, -496.4753680102650151 ) ) ;
#72994=CARTESIAN_POINT ( 'NONE',  ( -43.23652644599203398, -278.5081728373386341, -430.8702270131919363 ) ) ;
#72995=VECTOR ( 'NONE', #15811, 1000.000000000000000 ) ;
#73107=EDGE_CURVE ( 'NONE', #30245, #40166, #18706, .T. ) ;
#73156=CARTESIAN_POINT ( 'NONE',  ( -48.18343439339132317, -281.1256702228442350, -435.6442049081567234 ) ) ;
#73212=EDGE_LOOP ( 'NONE', ( #68515, #23371, #86569, #26362 ) ) ;
#73389=CARTESIAN_POINT ( 'NONE',  ( -48.18343439339133027, -259.3094209318401795, -498.0507307272308140 ) ) ;
#73618=CARTESIAN_POINT ( 'NONE',  ( -48.18343439339133027, -273.4097382619042378, -437.2279360942457060 ) ) ;
#73707=CARTESIAN_POINT ( 'NONE',  ( -48.18343439339133027, -268.0651010539349386, -439.6569430058891044 ) ) ;
#73887=ORIENTED_EDGE ( 'NONE', *, *, #3993, .T. ) ;
#73999=VERTEX_POINT ( 'NONE', #23858 ) ;
#74160=CARTESIAN_POINT ( 'NONE',  ( -48.18343439339133027, -268.4940904799746590, -439.4148130071812375 ) ) ;
#74180=CARTESIAN_POINT ( 'NONE',  ( -48.18343439339132317, -264.8229914578101329, -496.4753680103029296 ) ) ;
#74220=DIRECTION ( 'NONE',  ( -0.000000000000000000, 1.000000000000000000, 0.000000000000000000 ) ) ;
#74272=CYLINDRICAL_SURFACE ( 'NONE', #89641, 239.0731808058633874 ) ;
#74447=ORIENTED_EDGE ( 'NONE', *, *, #62145, .T. ) ;
#74599=CARTESIAN_POINT ( 'NONE',  ( -43.18343439339132317, -296.0521521680024080, -430.6442049081568939 ) ) ;
#74604=VECTOR ( 'NONE', #23250, 1000.000000000000000 ) ;
#74636=CARTESIAN_POINT ( 'NONE',  ( -48.18343439339133027, -261.1465603064251013, -445.1129026112485008 ) ) ;
#74868=ADVANCED_FACE ( 'NONE', ( #56504 ), #27132, .T. ) ;
#75105=CARTESIAN_POINT ( 'NONE',  ( -43.46159258565068484, -256.7356084326983137, -442.5391655924274801 ) ) ;
#75124=CARTESIAN_POINT ( 'NONE',  ( -48.18343439339133738, -271.8989017423947985, -505.6992907147873666 ) ) ;
#75126=CARTESIAN_POINT ( 'NONE',  ( -48.18343439339134449, -272.5190275734764782, -500.7427710990145329 ) ) ;
#75421=ORIENTED_EDGE ( 'NONE', *, *, #36276, .F. ) ;
#75449=SPHERICAL_SURFACE ( 'NONE', #48865, 35.00000000000000000 ) ;
#75562=CARTESIAN_POINT ( 'NONE',  ( -48.18343439337932210, -275.7009706631373547, -431.5134930252627896 ) ) ;
#75581=CARTESIAN_POINT ( 'NONE',  ( -48.18343439338108425, -263.3051960260782494, -501.2887401258802811 ) ) ;
#75726=CARTESIAN_POINT ( 'NONE',  ( -43.53359176515032658, -248.9304517128276473, -457.6964974781342335 ) ) ;
#76025=VECTOR ( 'NONE', #51232, 1000.000000000000000 ) ;
#76049=CARTESIAN_POINT ( 'NONE',  ( -43.27349326848973732, -275.1676604347916282, -506.7546311057413959 ) ) ;
#76118=CARTESIAN_POINT ( 'NONE',  ( -43.41266492080073647, -261.7876796617941295, -500.4428755130637683 ) ) ;
#76165=VECTOR ( 'NONE', #72754, 1000.000000000000000 ) ;
#76203=CARTESIAN_POINT ( 'NONE',  ( -48.18343439339133027, -254.4948186591712158, -445.8861037206912670 ) ) ;
#76311=FACE_OUTER_BOUND ( 'NONE', #19035, .T. ) ;
#76488=DIRECTION ( 'NONE',  ( 0.000000000000000000, 0.000000000000000000, 1.000000000000000000 ) ) ;
#76523=CARTESIAN_POINT ( 'NONE',  ( -43.52490746412112088, -249.8961441073384151, -483.9573757348985055 ) ) ;
#76589=CARTESIAN_POINT ( 'NONE',  ( -43.50899003844633484, -251.6488149788269197, -488.1642653036145703 ) ) ;
#76665=CARTESIAN_POINT ( 'NONE',  ( -48.18343439338449485, -249.5219462827487860, -456.6705712887342088 ) ) ;
#76860=ADVANCED_FACE ( 'NONE', ( #40040 ), #71805, .T. ) ;
#76939=ORIENTED_EDGE ( 'NONE', *, *, #42150, .T. ) ;
#77050=CIRCLE ( 'NONE', #31694, 5.000000000000004441 ) ;
#77051=CARTESIAN_POINT ( 'NONE',  ( -43.53958148833284270, -248.2611259770202139, -477.2465563938658306 ) ) ;
#77133=CARTESIAN_POINT ( 'NONE',  ( -48.18343439339133027, -254.0284636145295849, -457.8806065563774723 ) ) ;
#77324=EDGE_CURVE ( 'NONE', #41101, #42782, #32114, .T. ) ;
#77516=CARTESIAN_POINT ( 'NONE',  ( -48.18343439339133027, -291.0521521680024080, -435.6442049081568939 ) ) ;
#77718=DIRECTION ( 'NONE',  ( 0.000000000000000000, 0.000000000000000000, 1.000000000000000000 ) ) ;
#78399=ADVANCED_FACE ( 'NONE', ( #70721 ), #27627, .T. ) ;
#78706=CARTESIAN_POINT ( 'NONE',  ( -43.47537869213319084, -255.2745817066169423, -444.3374207175232868 ) ) ;
#78853=CARTESIAN_POINT ( 'NONE',  ( -48.18343439339133027, -261.1465603064058314, -445.1129026112122347 ) ) ;
#79055=CARTESIAN_POINT ( 'NONE',  ( -43.18343439339132317, -486.4924983417995463, -507.6442049081570076 ) ) ;
#79091=AXIS2_PLACEMENT_3D ( 'NONE', #1357, #88458, #39179 ) ;
#79113=FACE_OUTER_BOUND ( 'NONE', #24982, .T. ) ;
#79241=CIRCLE ( 'NONE', #14230, 35.00000000000003553 ) ;
#79758=DIRECTION ( 'NONE',  ( 1.000000000000000000, 0.000000000000000000, 0.000000000000000000 ) ) ;
#79871=CARTESIAN_POINT ( 'NONE',  ( 41.08708295871279859, -293.9068999365417199, -472.6442049081569508 ) ) ;
#79937=DIRECTION ( 'NONE',  ( 0.000000000000000000, 0.000000000000000000, 1.000000000000000000 ) ) ;
#79960=CARTESIAN_POINT ( 'NONE',  ( -43.18343439339132317, -296.0521521680024080, -430.6442049081568939 ) ) ;
#80012=CARTESIAN_POINT ( 'NONE',  ( -43.49048823363975202, -253.6564221937692594, -491.6618016576409218 ) ) ;
#80092=CARTESIAN_POINT ( 'NONE',  ( -43.54160339317392214, -248.0334966641272842, -465.6442049081569508 ) ) ;
#80464=CARTESIAN_POINT ( 'NONE',  ( -43.21050657630429015, -280.7973232067119511, -507.6442049081570076 ) ) ;
#80785=LINE ( 'NONE', #87864, #76165 ) ;
#80841=DIRECTION ( 'NONE',  ( 0.000000000000000000, 0.000000000000000000, 1.000000000000000000 ) ) ;
#80868=EDGE_LOOP ( 'NONE', ( #66667, #30185, #52012, #76939 ) ) ;
#80940=CARTESIAN_POINT ( 'NONE',  ( -48.18343439339133027, -281.1256972089279884, -502.6442049077165279 ) ) ;
#81057=CARTESIAN_POINT ( 'NONE',  ( 76.08708295871279859, -296.0521521680024080, -465.6442049081569508 ) ) ;
#81121=ORIENTED_EDGE ( 'NONE', *, *, #22861, .T. ) ;
#81259=CARTESIAN_POINT ( 'NONE',  ( -48.18343439339133027, -267.2165102599228135, -440.1639404234281301 ) ) ;
#81279=CARTESIAN_POINT ( 'NONE',  ( -48.18343439339131606, -257.5766546844495792, -488.5262689091994730 ) ) ;
#81317=FACE_OUTER_BOUND ( 'NONE', #19519, .T. ) ;
#81351=ORIENTED_EDGE ( 'NONE', *, *, #42527, .F. ) ;
#81359=AXIS2_PLACEMENT_3D ( 'NONE', #26799, #5961, #12597 ) ;
#81368=ADVANCED_FACE ( 'NONE', ( #79113 ), #14261, .T. ) ;
#81609=CARTESIAN_POINT ( 'NONE',  ( 52.66432107828247666, -260.8771019122912094, -472.6442049081569508 ) ) ;
#81718=CARTESIAN_POINT ( 'NONE',  ( -48.18343439339133027, -274.8200403470382298, -436.8002545823482023 ) ) ;
#81739=CARTESIAN_POINT ( 'NONE',  ( -48.18343439339132317, -257.8434817577606282, -488.9450021220059170 ) ) ;
#81759=CARTESIAN_POINT ( 'NONE',  ( 41.08708295871279859, -296.0521521680024080, -472.6442049081569508 ) ) ;
#81847=DIRECTION ( 'NONE',  ( -0.9437085149785860994, 0.3307782319877048405, 0.000000000000000000 ) ) ;
#82195=CARTESIAN_POINT ( 'NONE',  ( -43.37475307536850266, -265.5729591849662938, -435.3257326888780199 ) ) ;
#82236=DIRECTION ( 'NONE',  ( -0.3307782319877045629, -0.9437085149785860994, 0.000000000000000000 ) ) ;
#82387=SHAPE_DEFINITION_REPRESENTATION ( #48138, #30030 ) ;
#82638=FACE_OUTER_BOUND ( 'NONE', #66434, .T. ) ;
#82656=CARTESIAN_POINT ( 'NONE',  ( -48.18343439339133027, -276.2535042660651925, -436.4286699060542674 ) ) ;
#82676=CARTESIAN_POINT ( 'NONE',  ( -48.18343439339132317, -270.8128065642191018, -505.3008612166128728 ) ) ;
#82739=CARTESIAN_POINT ( 'NONE',  ( -43.43031340896369130, -259.9895260090733586, -498.9919023260428048 ) ) ;
#82802=ORIENTED_EDGE ( 'NONE', *, *, #8182, .T. ) ;
#82819=CARTESIAN_POINT ( 'NONE',  ( -48.18343439339133027, -254.9491769968546464, -455.0632279659918140 ) ) ;
#83115=CARTESIAN_POINT ( 'NONE',  ( -43.47198418667934305, -255.6354909541967970, -443.8759249308465655 ) ) ;
#83132=CARTESIAN_POINT ( 'NONE',  ( -43.35434167168779851, -267.5826604045195154, -504.1128848280075090 ) ) ;
#83134=CARTESIAN_POINT ( 'NONE',  ( -48.18343439339133738, -255.2824783920493132, -484.1824042360379394 ) ) ;
#83164=UNCERTAINTY_MEASURE_WITH_UNIT (LENGTH_MEASURE( 1.000000000000000082E-05 ), #18050, 'distance_accuracy_value', 'NONE');
#83215=EDGE_CURVE ( 'NONE', #30930, #34997, #68628, .T. ) ;
#83282=DIRECTION ( 'NONE',  ( -1.000000000000000000, 0.000000000000000000, 0.000000000000000000 ) ) ;
#83295=ORIENTED_EDGE ( 'NONE', *, *, #59476, .T. ) ;
#83488=EDGE_CURVE ( 'NONE', #73999, #2981, #24763, .T. ) ;
#83599=CARTESIAN_POINT ( 'NONE',  ( -48.18343439339133027, -256.1235685799528596, -485.9512705678166640 ) ) ;
#83748=AXIS2_PLACEMENT_3D ( 'NONE', #81759, #44383, #80841 ) ;
#83986=EDGE_CURVE ( 'NONE', #58159, #40166, #44418, .T. ) ;
#84021=ORIENTED_EDGE ( 'NONE', *, *, #77324, .F. ) ;
#84073=CARTESIAN_POINT ( 'NONE',  ( -43.52140980873610943, -250.2833644051135593, -485.0314067457711076 ) ) ;
#84139=CARTESIAN_POINT ( 'NONE',  ( -43.49340244127498067, -253.3420193263868896, -491.1679700123006569 ) ) ;
#84219=CARTESIAN_POINT ( 'NONE',  ( -48.18343439339133027, -258.3625464905638296, -448.5700876443999050 ) ) ;
#84263=DIRECTION ( 'NONE',  ( 1.000000000000000000, 0.000000000000000000, 0.000000000000000000 ) ) ;
#84535=CARTESIAN_POINT ( 'NONE',  ( -48.18343439339132317, -253.0206516614774728, -472.6442049081569508 ) ) ;
#85006=CARTESIAN_POINT ( 'NONE',  ( -48.18343439339133027, -248.3668650810686529, -472.6442049081570076 ) ) ;
#85656=ADVANCED_FACE ( 'NONE', ( #76311 ), #11902, .F. ) ;
#85701=FACE_OUTER_BOUND ( 'NONE', #73212, .T. ) ;
#85820=DIRECTION ( 'NONE',  ( 0.000000000000000000, 1.000000000000000000, 0.000000000000000000 ) ) ;
#85867=ORIENTED_EDGE ( 'NONE', *, *, #43526, .T. ) ;
#85941=CARTESIAN_POINT ( 'NONE',  ( -48.18343439339133027, -254.6019642153539735, -455.9944935231090994 ) ) ;
#86004=CARTESIAN_POINT ( 'NONE',  ( -48.18343439339133027, -291.0521521680024080, -430.6442049081568939 ) ) ;
#86280=CARTESIAN_POINT ( 'NONE',  ( 41.08708295871279859, -293.9068999365417199, -465.6442049081569508 ) ) ;
#86528=VERTEX_POINT ( 'NONE', #17513 ) ;
#86569=ORIENTED_EDGE ( 'NONE', *, *, #68922, .F. ) ;
#86594=LINE ( 'NONE', #79055, #32229 ) ;
#86720=CARTESIAN_POINT ( 'NONE',  ( -43.38975745197526379, -264.0880790402558773, -436.2305102663831349 ) ) ;
#86729=AXIS2_PLACEMENT_3D ( 'NONE', #2709, #89316, #82236 ) ;
#87184=CARTESIAN_POINT ( 'NONE',  ( -43.29223561230568151, -273.4430627291207543, -431.9941326777201880 ) ) ;
#87518=VERTEX_POINT ( 'NONE', #77516 ) ;
#87558=CARTESIAN_POINT ( 'NONE',  ( -48.18343439339133027, -253.5923708015767772, -491.0188676228033273 ) ) ;
#87569=VECTOR ( 'NONE', #66402, 1000.000000000000000 ) ;
#87600=ORIENTED_EDGE ( 'NONE', *, *, #64244, .T. ) ;
#87640=CARTESIAN_POINT ( 'NONE',  ( -43.18343439339132317, -283.1093320178187582, -430.6442049081568939 ) ) ;
#87794=CARTESIAN_POINT ( 'NONE',  ( -48.18343439339132317, -253.7899642232643203, -458.8318842538539002 ) ) ;
#87864=CARTESIAN_POINT ( 'NONE',  ( 76.08708295871279859, -293.9068999365417199, -430.6442049081568939 ) ) ;
#88019=CARTESIAN_POINT ( 'NONE',  ( -48.18343439339133027, -272.5190275734900069, -500.7427710989320531 ) ) ;
#88022=PLANE ( 'NONE',  #55166 ) ;
#88107=( GEOMETRIC_REPRESENTATION_CONTEXT ( 3 ) GLOBAL_UNCERTAINTY_ASSIGNED_CONTEXT ( ( #83164 ) ) GLOBAL_UNIT_ASSIGNED_CONTEXT ( ( #18050, #39795, #31789 ) ) REPRESENTATION_CONTEXT ( 'NONE', 'WORKASPACE' ) );
#88166=AXIS2_PLACEMENT_3D ( 'NONE', #10891, #47808, #55877 ) ;
#88266=AXIS2_PLACEMENT_3D ( 'NONE', #26556, #34133, #11407 ) ;
#88338=PLANE ( 'NONE',  #42628 ) ;
#88458=DIRECTION ( 'NONE',  ( 0.000000000000000000, 0.000000000000000000, 1.000000000000000000 ) ) ;
#88552=ORIENTED_EDGE ( 'NONE', *, *, #37852, .T. ) ;
#88787=LINE ( 'NONE', #74599, #19011 ) ;
#88819=CARTESIAN_POINT ( 'NONE',  ( -48.18343439339133027, -260.4846106489175668, -445.8398854946390202 ) ) ;
#88909=PLANE ( 'NONE',  #79091 ) ;
#89245=VERTEX_POINT ( 'NONE', #10296 ) ;
#89277=CARTESIAN_POINT ( 'NONE',  ( -43.32131299890800591, -270.7287516391538134, -432.8764281593785199 ) ) ;
#89296=CARTESIAN_POINT ( 'NONE',  ( -48.18343439339133027, -253.0206516614774728, -472.6442049081569508 ) ) ;
#89316=DIRECTION ( 'NONE',  ( -0.9437085149785860994, 0.3307782319877048405, 0.000000000000000000 ) ) ;
#89366=ADVANCED_FACE ( 'NONE', ( #33020 ), #18346, .T. ) ;
#89532=ORIENTED_EDGE ( 'NONE', *, *, #28676, .F. ) ;
#89613=DIRECTION ( 'NONE',  ( -0.000000000000000000, -1.000000000000000000, -0.000000000000000000 ) ) ;
#89641=AXIS2_PLACEMENT_3D ( 'NONE', #67192, #44459, #45848 ) ;
#89751=CARTESIAN_POINT ( 'NONE',  ( -48.18343439339133027, -264.2011365548906383, -436.3931507628129225 ) ) ;
#89769=CARTESIAN_POINT ( 'NONE',  ( -43.23635059700391992, -278.5233168282929910, -507.4184232499240466 ) ) ;
#89771=CARTESIAN_POINT ( 'NONE',  ( -48.18343439339134449, -259.2200010662057821, -490.9919136893941527 ) ) ;
#89789=AXIS2_PLACEMENT_3D ( 'NONE', #40003, #76488, #46181 ) ;
#89840=CARTESIAN_POINT ( 'NONE',  ( -43.35439945481423507, -267.5770695277309983, -504.1101809961486993 ) ) ;
#90216=CARTESIAN_POINT ( 'NONE',  ( -48.18343439338967471, -273.4767344845260482, -432.0952024610487001 ) ) ;
#90233=CARTESIAN_POINT ( 'NONE',  ( -48.18343439339133027, -275.3442733027022200, -501.6452696258747324 ) ) ;
#90235=CARTESIAN_POINT ( 'NONE',  ( -48.18343439339132317, -275.3442733027010831, -501.6452696257773596 ) ) ;
#90375=CARTESIAN_POINT ( 'NONE',  ( -43.51953433940560956, -250.4898501243895055, -452.7628537496786407 ) ) ;
#90531=DIRECTION ( 'NONE',  ( 0.000000000000000000, 0.000000000000000000, 1.000000000000000000 ) ) ;
#90750=CARTESIAN_POINT ( 'NONE',  ( -43.49052031076330138, -253.6529657927480343, -491.6564673409728243 ) ) ;
#90831=CARTESIAN_POINT ( 'NONE',  ( -48.18343439339476220, -250.0149903365356749, -455.0345092807172023 ) ) ;
#90959=CARTESIAN_POINT ( 'NONE',  ( 0.000000000000000000, 0.000000000000000000, 0.000000000000000000 ) ) ;
#91011=EDGE_CURVE ( 'NONE', #58102, #89245, #88787, .T. ) ;
#91022=DIRECTION ( 'NONE',  ( 0.000000000000000000, -1.000000000000000000, 0.000000000000000000 ) ) ;
#91231=CARTESIAN_POINT ( 'NONE',  ( -43.28564603558642432, -274.0543938782848272, -506.4777364308019401 ) ) ;
#91317=CARTESIAN_POINT ( 'NONE',  ( -48.18343439339133027, -254.6143759403197180, -455.9956540770752440 ) ) ;
#91371=CARTESIAN_POINT ( 'NONE',  ( 41.08708295871279859, -293.9068999365417199, -430.6442049081568939 ) ) ;
#91644=CARTESIAN_POINT ( 'NONE',  ( -43.53335306050103526, -248.9569719664657157, -480.6442262660607980 ) ) ;
#91721=CARTESIAN_POINT ( 'NONE',  ( -48.18343439339133027, -283.5835610574164889, -435.6442049081568939 ) ) ;
#91790=CARTESIAN_POINT ( 'NONE',  ( -43.47533972853607054, -255.2787295525174613, -444.3320233189222677 ) ) ;
#91968=ADVANCED_FACE ( 'NONE', ( #57711 ), #29640, .T. ) ;
#92088=DIRECTION ( 'NONE',  ( -0.000000000000000000, 1.000000000000000000, 0.000000000000000000 ) ) ;
#92110=CARTESIAN_POINT ( 'NONE',  ( -43.52943240505717171, -249.3936360501505476, -482.3142747188312569 ) ) ;
#92450=DIRECTION ( 'NONE',  ( 1.000000000000000000, 0.000000000000000000, 0.000000000000000000 ) ) ;
#92576=AXIS2_PLACEMENT_3D ( 'NONE', #86280, #85820, #49838 ) ;
#93012=EDGE_LOOP ( 'NONE', ( #49071, #19376, #17538 ) ) ;
#93057=CARTESIAN_POINT ( 'NONE',  ( -48.18343439339133738, -253.0206516614774728, -463.6603765730280315 ) ) ;
#93190=DIRECTION ( 'NONE',  ( -0.000000000000000000, -0.000000000000000000, -1.000000000000000000 ) ) ;
#93366=CARTESIAN_POINT ( 'NONE',  ( -43.27403345252375289, -275.1145486516829237, -431.5602653418008003 ) ) ;
#93689=DIRECTION ( 'NONE',  ( 1.000000000000000000, 0.000000000000000000, 0.000000000000000000 ) ) ;
#93732=COLOUR_RGB('Light Blue',0.38,0.62,0.78);
#93733=FILL_AREA_STYLE_COLOUR('',#93732);
#93734=FILL_AREA_STYLE('',(#93733));
#93735=SURFACE_STYLE_FILL_AREA(#93734);
#93736=SURFACE_SIDE_STYLE('',(#93735));
#93737=SURFACE_STYLE_USAGE(.BOTH.,#93736);
#93738=PRESENTATION_STYLE_ASSIGNMENT((#93737));
ENDSEC;
END-ISO-10303-21;
